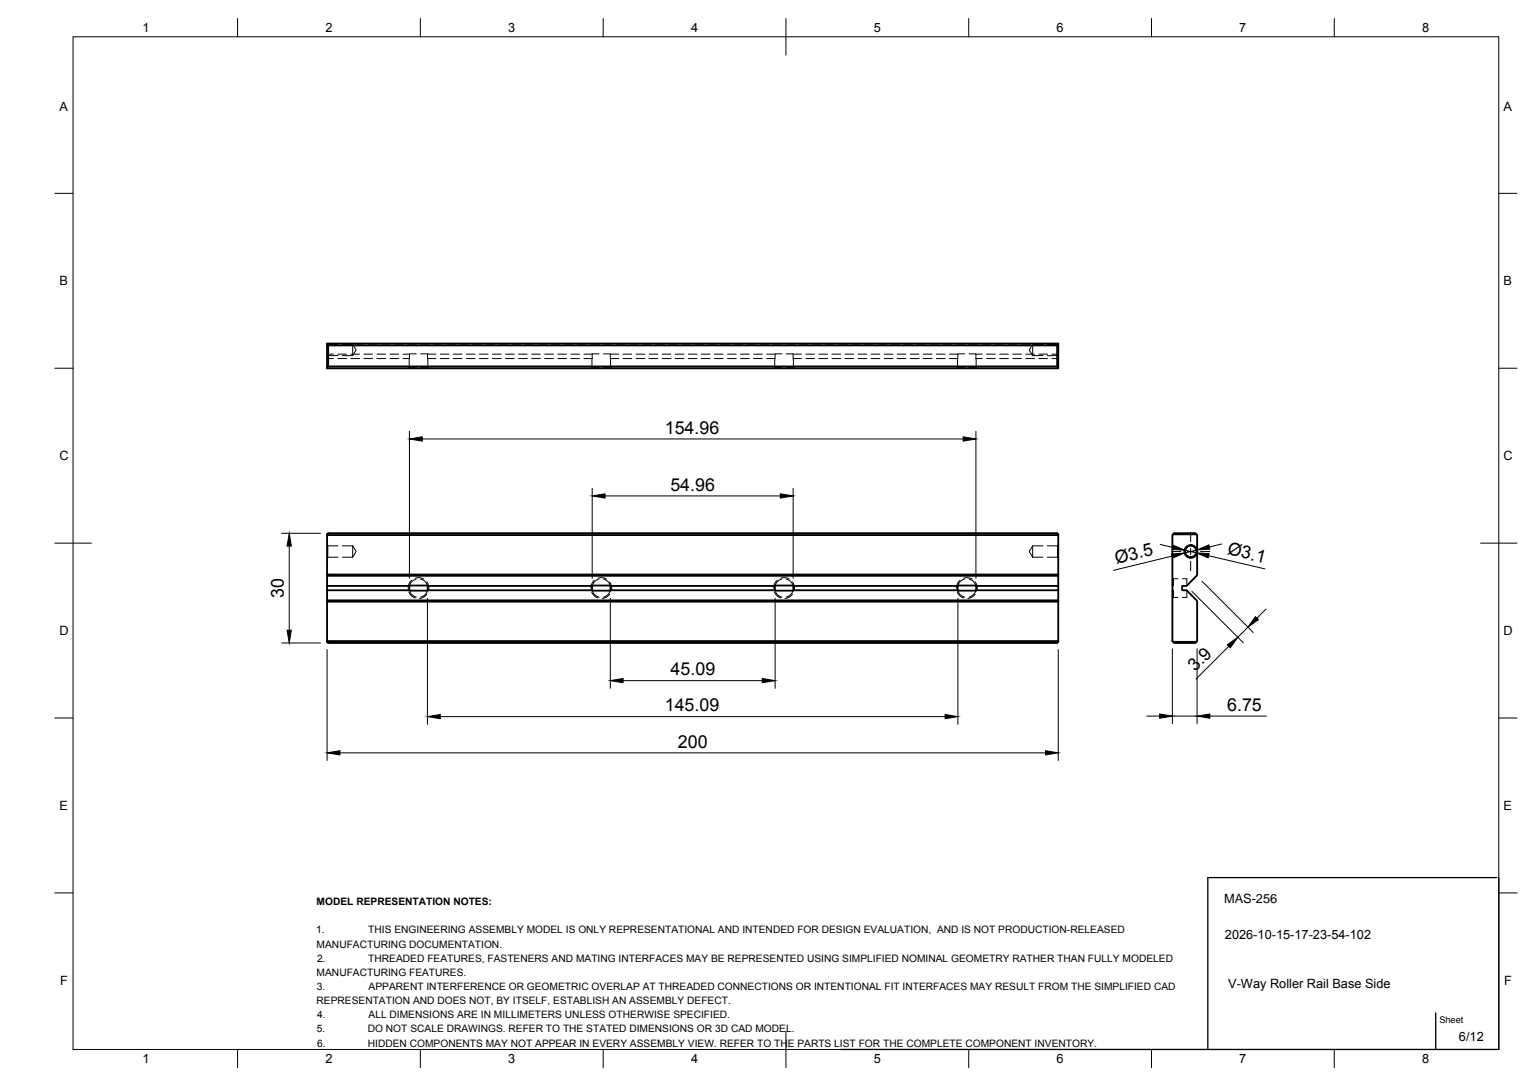
ISO-10303-21;
HEADER;
/* Generated by software containing ST-Developer
 * from STEP Tools, Inc. (www.steptools.com) 
 */

FILE_DESCRIPTION(
/* description */ (''),
/* implementation_level */ '2;1');

FILE_NAME(
/* name */ 'V-Way Roller Rail Base Side.step',
/* time_stamp */ '2026-10-14T18:40:07-07:00',
/* author */ (''),
/* organization */ (''),
/* preprocessor_version */ 'ST-DEVELOPER v20.2',
/* originating_system */ 'Autodesk Translation Framework v15.15.0.0',
/* authorisation */ '');

FILE_SCHEMA (('AUTOMOTIVE_DESIGN { 1 0 10303 214 3 1 1 }'));
ENDSEC;

DATA;
#10=MECHANICAL_DESIGN_GEOMETRIC_PRESENTATION_REPRESENTATION('',(#834),#81040);
#384=ELLIPSE('',#15733,3.60624458405138,2.54999999999999);
#385=ELLIPSE('',#15735,3.60624458405138,2.54999999999999);
#386=ELLIPSE('',#15737,3.60624458405138,2.54999999999999);
#387=ELLIPSE('',#15739,3.60624458405138,2.54999999999999);
#388=ELLIPSE('',#15745,3.60624458405139,2.55);
#389=ELLIPSE('',#15747,3.60624458405139,2.55);
#390=ELLIPSE('',#15749,3.60624458405139,2.55);
#391=ELLIPSE('',#15751,3.60624458405139,2.55);
#392=ELLIPSE('',#15757,3.60624458405141,2.55000000000001);
#393=ELLIPSE('',#15759,3.60624458405141,2.55000000000001);
#394=ELLIPSE('',#15761,3.6062445840514,2.55000000000001);
#395=ELLIPSE('',#15763,3.6062445840514,2.55000000000001);
#396=ELLIPSE('',#15769,3.60624458405141,2.55000000000001);
#397=ELLIPSE('',#15771,3.60624458405141,2.55000000000001);
#398=ELLIPSE('',#15773,3.6062445840514,2.55000000000001);
#399=ELLIPSE('',#15775,3.6062445840514,2.55000000000001);
#814=SHAPE_REPRESENTATION_RELATIONSHIP('SRR','None',#81133,#824);
#824=ADVANCED_BREP_SHAPE_REPRESENTATION('',(#844),#81033);
#834=STYLED_ITEM('',(#81192),#844);
#844=MANIFOLD_SOLID_BREP('Body1',#15087);
#920=CYLINDRICAL_SURFACE('',#15711,1.55);
#921=CYLINDRICAL_SURFACE('',#15720,1.55);
#922=CYLINDRICAL_SURFACE('',#15731,2.54999999999999);
#923=CYLINDRICAL_SURFACE('',#15743,2.55);
#924=CYLINDRICAL_SURFACE('',#15755,2.55000000000001);
#925=CYLINDRICAL_SURFACE('',#15767,2.55000000000001);
#1172=FACE_BOUND('',#2705,.T.);
#1173=FACE_BOUND('',#2706,.T.);
#1174=FACE_BOUND('',#2707,.T.);
#1175=FACE_BOUND('',#2708,.T.);
#1320=PLANE('',#15710);
#1321=PLANE('',#15719);
#1322=PLANE('',#15727);
#1323=PLANE('',#15777);
#1324=PLANE('',#15778);
#1325=PLANE('',#15779);
#1326=PLANE('',#15780);
#1327=PLANE('',#15781);
#1328=PLANE('',#15782);
#1329=PLANE('',#15783);
#1330=PLANE('',#15784);
#1331=PLANE('',#15785);
#1332=PLANE('',#15786);
#1333=PLANE('',#15787);
#1334=PLANE('',#15788);
#1335=PLANE('',#15789);
#1336=PLANE('',#15790);
#1337=PLANE('',#15791);
#1338=PLANE('',#15792);
#1339=PLANE('',#15793);
#1340=PLANE('',#15794);
#1341=PLANE('',#15795);
#1342=PLANE('',#15796);
#1343=PLANE('',#15797);
#1344=PLANE('',#15798);
#1345=PLANE('',#15799);
#1346=PLANE('',#15800);
#1347=PLANE('',#15801);
#1348=PLANE('',#15802);
#1349=PLANE('',#15803);
#1350=PLANE('',#15804);
#1351=PLANE('',#15805);
#1352=PLANE('',#15806);
#1353=PLANE('',#15807);
#1354=PLANE('',#15808);
#1355=PLANE('',#15809);
#1356=PLANE('',#15810);
#1357=PLANE('',#15811);
#1358=PLANE('',#15812);
#1359=PLANE('',#15813);
#1360=PLANE('',#15814);
#1361=PLANE('',#15815);
#1863=FACE_OUTER_BOUND('',#2695,.T.);
#1864=FACE_OUTER_BOUND('',#2696,.T.);
#1865=FACE_OUTER_BOUND('',#2697,.T.);
#1866=FACE_OUTER_BOUND('',#2698,.T.);
#1867=FACE_OUTER_BOUND('',#2699,.T.);
#1868=FACE_OUTER_BOUND('',#2700,.T.);
#1869=FACE_OUTER_BOUND('',#2701,.T.);
#1870=FACE_OUTER_BOUND('',#2702,.T.);
#1871=FACE_OUTER_BOUND('',#2703,.T.);
#1872=FACE_OUTER_BOUND('',#2704,.T.);
#1873=FACE_OUTER_BOUND('',#2709,.T.);
#1874=FACE_OUTER_BOUND('',#2710,.T.);
#1875=FACE_OUTER_BOUND('',#2711,.T.);
#1876=FACE_OUTER_BOUND('',#2712,.T.);
#1877=FACE_OUTER_BOUND('',#2713,.T.);
#1878=FACE_OUTER_BOUND('',#2714,.T.);
#1879=FACE_OUTER_BOUND('',#2715,.T.);
#1880=FACE_OUTER_BOUND('',#2716,.T.);
#1881=FACE_OUTER_BOUND('',#2717,.T.);
#1882=FACE_OUTER_BOUND('',#2718,.T.);
#1883=FACE_OUTER_BOUND('',#2719,.T.);
#1884=FACE_OUTER_BOUND('',#2720,.T.);
#1885=FACE_OUTER_BOUND('',#2721,.T.);
#1886=FACE_OUTER_BOUND('',#2722,.T.);
#1887=FACE_OUTER_BOUND('',#2723,.T.);
#1888=FACE_OUTER_BOUND('',#2724,.T.);
#1889=FACE_OUTER_BOUND('',#2725,.T.);
#1890=FACE_OUTER_BOUND('',#2726,.T.);
#1891=FACE_OUTER_BOUND('',#2727,.T.);
#1892=FACE_OUTER_BOUND('',#2728,.T.);
#1893=FACE_OUTER_BOUND('',#2729,.T.);
#1894=FACE_OUTER_BOUND('',#2730,.T.);
#1895=FACE_OUTER_BOUND('',#2731,.T.);
#1896=FACE_OUTER_BOUND('',#2732,.T.);
#1897=FACE_OUTER_BOUND('',#2733,.T.);
#1898=FACE_OUTER_BOUND('',#2734,.T.);
#1899=FACE_OUTER_BOUND('',#2735,.T.);
#1900=FACE_OUTER_BOUND('',#2736,.T.);
#1901=FACE_OUTER_BOUND('',#2737,.T.);
#1902=FACE_OUTER_BOUND('',#2738,.T.);
#1903=FACE_OUTER_BOUND('',#2739,.T.);
#1904=FACE_OUTER_BOUND('',#2740,.T.);
#1905=FACE_OUTER_BOUND('',#2741,.T.);
#1906=FACE_OUTER_BOUND('',#2742,.T.);
#1907=FACE_OUTER_BOUND('',#2743,.T.);
#1908=FACE_OUTER_BOUND('',#2744,.T.);
#1909=FACE_OUTER_BOUND('',#2745,.T.);
#1910=FACE_OUTER_BOUND('',#2746,.T.);
#1911=FACE_OUTER_BOUND('',#2747,.T.);
#1912=FACE_OUTER_BOUND('',#2748,.T.);
#1913=FACE_OUTER_BOUND('',#2749,.T.);
#1914=FACE_OUTER_BOUND('',#2750,.T.);
#1915=FACE_OUTER_BOUND('',#2751,.T.);
#1916=FACE_OUTER_BOUND('',#2752,.T.);
#1917=FACE_OUTER_BOUND('',#2753,.T.);
#1918=FACE_OUTER_BOUND('',#2754,.T.);
#2695=EDGE_LOOP('',(#11060,#11061,#11062,#11063,#11064));
#2696=EDGE_LOOP('',(#11065,#11066,#11067,#11068,#11069,#11070,#11071,#11072,
#11073,#11074,#11075,#11076,#11077,#11078,#11079,#11080,#11081,#11082,#11083));
#2697=EDGE_LOOP('',(#11084,#11085,#11086,#11087,#11088));
#2698=EDGE_LOOP('',(#11089,#11090,#11091,#11092));
#2699=EDGE_LOOP('',(#11093,#11094,#11095,#11096,#11097));
#2700=EDGE_LOOP('',(#11098,#11099,#11100,#11101,#11102,#11103,#11104,#11105,
#11106,#11107,#11108,#11109,#11110,#11111,#11112,#11113,#11114,#11115,#11116));
#2701=EDGE_LOOP('',(#11117,#11118,#11119,#11120,#11121));
#2702=EDGE_LOOP('',(#11122,#11123,#11124,#11125));
#2703=EDGE_LOOP('',(#11126,#11127,#11128,#11129));
#2704=EDGE_LOOP('',(#11130,#11131,#11132,#11133));
#2705=EDGE_LOOP('',(#11134));
#2706=EDGE_LOOP('',(#11135));
#2707=EDGE_LOOP('',(#11136));
#2708=EDGE_LOOP('',(#11137));
#2709=EDGE_LOOP('',(#11138,#11139,#11140,#11141,#11142,#11143,#11144,#11145,
#11146,#11147,#11148,#11149,#11150,#11151,#11152,#11153));
#2710=EDGE_LOOP('',(#11154,#11155,#11156,#11157));
#2711=EDGE_LOOP('',(#11158,#11159,#11160,#11161,#11162,#11163,#11164,#11165,
#11166,#11167,#11168,#11169,#11170,#11171,#11172,#11173));
#2712=EDGE_LOOP('',(#11174,#11175,#11176,#11177));
#2713=EDGE_LOOP('',(#11178,#11179,#11180,#11181,#11182,#11183,#11184,#11185,
#11186,#11187,#11188,#11189,#11190,#11191,#11192,#11193));
#2714=EDGE_LOOP('',(#11194,#11195,#11196,#11197));
#2715=EDGE_LOOP('',(#11198,#11199,#11200,#11201,#11202,#11203,#11204,#11205,
#11206,#11207,#11208,#11209,#11210,#11211,#11212,#11213));
#2716=EDGE_LOOP('',(#11214,#11215));
#2717=EDGE_LOOP('',(#11216,#11217));
#2718=EDGE_LOOP('',(#11218,#11219));
#2719=EDGE_LOOP('',(#11220,#11221));
#2720=EDGE_LOOP('',(#11222,#11223));
#2721=EDGE_LOOP('',(#11224,#11225));
#2722=EDGE_LOOP('',(#11226,#11227));
#2723=EDGE_LOOP('',(#11228,#11229));
#2724=EDGE_LOOP('',(#11230,#11231,#11232,#11233,#11234,#11235,#11236,#11237,
#11238,#11239,#11240,#11241,#11242,#11243,#11244,#11245,#11246,#11247,#11248,
#11249));
#2725=EDGE_LOOP('',(#11250,#11251,#11252,#11253));
#2726=EDGE_LOOP('',(#11254,#11255,#11256,#11257));
#2727=EDGE_LOOP('',(#11258,#11259,#11260,#11261));
#2728=EDGE_LOOP('',(#11262,#11263,#11264,#11265));
#2729=EDGE_LOOP('',(#11266,#11267,#11268,#11269));
#2730=EDGE_LOOP('',(#11270,#11271,#11272,#11273,#11274));
#2731=EDGE_LOOP('',(#11275,#11276,#11277,#11278,#11279));
#2732=EDGE_LOOP('',(#11280,#11281,#11282,#11283,#11284));
#2733=EDGE_LOOP('',(#11285,#11286,#11287,#11288));
#2734=EDGE_LOOP('',(#11289,#11290,#11291,#11292));
#2735=EDGE_LOOP('',(#11293,#11294,#11295,#11296));
#2736=EDGE_LOOP('',(#11297,#11298,#11299,#11300));
#2737=EDGE_LOOP('',(#11301,#11302,#11303,#11304));
#2738=EDGE_LOOP('',(#11305,#11306,#11307,#11308,#11309,#11310));
#2739=EDGE_LOOP('',(#11311,#11312,#11313,#11314));
#2740=EDGE_LOOP('',(#11315,#11316,#11317,#11318,#11319,#11320));
#2741=EDGE_LOOP('',(#11321,#11322,#11323,#11324));
#2742=EDGE_LOOP('',(#11325,#11326,#11327,#11328));
#2743=EDGE_LOOP('',(#11329,#11330,#11331,#11332));
#2744=EDGE_LOOP('',(#11333,#11334,#11335,#11336));
#2745=EDGE_LOOP('',(#11337,#11338,#11339,#11340));
#2746=EDGE_LOOP('',(#11341,#11342,#11343,#11344,#11345,#11346,#11347,#11348,
#11349,#11350,#11351,#11352,#11353,#11354,#11355,#11356,#11357,#11358,#11359,
#11360));
#2747=EDGE_LOOP('',(#11361,#11362,#11363,#11364));
#2748=EDGE_LOOP('',(#11365,#11366,#11367,#11368,#11369,#11370));
#2749=EDGE_LOOP('',(#11371,#11372,#11373,#11374,#11375,#11376));
#2750=EDGE_LOOP('',(#11377,#11378,#11379,#11380,#11381,#11382));
#2751=EDGE_LOOP('',(#11383,#11384,#11385,#11386));
#2752=EDGE_LOOP('',(#11387,#11388,#11389,#11390));
#2753=EDGE_LOOP('',(#11391,#11392,#11393,#11394,#11395));
#2754=EDGE_LOOP('',(#11396,#11397,#11398,#11399));
#3614=LINE('',#21912,#4726);
#3615=LINE('',#21919,#4727);
#3616=LINE('',#21921,#4728);
#3617=LINE('',#21923,#4729);
#3618=LINE('',#21925,#4730);
#3619=LINE('',#21927,#4731);
#3620=LINE('',#21929,#4732);
#3621=LINE('',#21931,#4733);
#3622=LINE('',#21933,#4734);
#3623=LINE('',#21935,#4735);
#3624=LINE('',#21937,#4736);
#3625=LINE('',#21938,#4737);
#3626=LINE('',#21940,#4738);
#3627=LINE('',#21942,#4739);
#3628=LINE('',#21944,#4740);
#3629=LINE('',#21946,#4741);
#3630=LINE('',#21948,#4742);
#3631=LINE('',#21949,#4743);
#3632=LINE('',#21952,#4744);
#3633=LINE('',#21958,#4745);
#3634=LINE('',#21963,#4746);
#3635=LINE('',#21970,#4747);
#3636=LINE('',#21972,#4748);
#3637=LINE('',#21973,#4749);
#3638=LINE('',#21975,#4750);
#3639=LINE('',#21977,#4751);
#3640=LINE('',#21979,#4752);
#3641=LINE('',#21981,#4753);
#3642=LINE('',#21983,#4754);
#3643=LINE('',#21985,#4755);
#3644=LINE('',#21987,#4756);
#3645=LINE('',#21989,#4757);
#3646=LINE('',#21991,#4758);
#3647=LINE('',#21993,#4759);
#3648=LINE('',#21995,#4760);
#3649=LINE('',#21997,#4761);
#3650=LINE('',#21999,#4762);
#3651=LINE('',#22000,#4763);
#3652=LINE('',#22003,#4764);
#3653=LINE('',#22009,#4765);
#3654=LINE('',#22014,#4766);
#3655=LINE('',#22017,#4767);
#3656=LINE('',#22018,#4768);
#3657=LINE('',#22027,#4769);
#3658=LINE('',#22031,#4770);
#3659=LINE('',#22039,#4771);
#3660=LINE('',#22043,#4772);
#3661=LINE('',#22051,#4773);
#3662=LINE('',#22056,#4774);
#3663=LINE('',#22059,#4775);
#3664=LINE('',#22063,#4776);
#3665=LINE('',#22071,#4777);
#3666=LINE('',#22075,#4778);
#3667=LINE('',#22083,#4779);
#3668=LINE('',#22088,#4780);
#3669=LINE('',#22091,#4781);
#3670=LINE('',#22095,#4782);
#3671=LINE('',#22103,#4783);
#3672=LINE('',#22107,#4784);
#3673=LINE('',#22115,#4785);
#3674=LINE('',#22120,#4786);
#3675=LINE('',#22123,#4787);
#3676=LINE('',#22127,#4788);
#3677=LINE('',#22135,#4789);
#3678=LINE('',#22139,#4790);
#3679=LINE('',#22147,#4791);
#3680=LINE('',#22150,#4792);
#3681=LINE('',#22152,#4793);
#3682=LINE('',#22154,#4794);
#3683=LINE('',#22156,#4795);
#3684=LINE('',#22158,#4796);
#3685=LINE('',#22160,#4797);
#3686=LINE('',#22162,#4798);
#3687=LINE('',#22164,#4799);
#3688=LINE('',#22166,#4800);
#3689=LINE('',#22167,#4801);
#3690=LINE('',#22168,#4802);
#3691=LINE('',#22169,#4803);
#3692=LINE('',#22170,#4804);
#3693=LINE('',#22171,#4805);
#3694=LINE('',#22173,#4806);
#3695=LINE('',#22175,#4807);
#3696=LINE('',#22177,#4808);
#3697=LINE('',#22179,#4809);
#3698=LINE('',#22181,#4810);
#3699=LINE('',#22183,#4811);
#3700=LINE('',#22185,#4812);
#3701=LINE('',#22187,#4813);
#3702=LINE('',#22189,#4814);
#3703=LINE('',#22191,#4815);
#3704=LINE('',#22193,#4816);
#3705=LINE('',#22195,#4817);
#3706=LINE('',#22198,#4818);
#3707=LINE('',#22200,#4819);
#3708=LINE('',#22201,#4820);
#3709=LINE('',#22204,#4821);
#3710=LINE('',#22205,#4822);
#3711=LINE('',#22208,#4823);
#3712=LINE('',#22210,#4824);
#3713=LINE('',#22211,#4825);
#3714=LINE('',#22214,#4826);
#3715=LINE('',#22215,#4827);
#3716=LINE('',#22218,#4828);
#3717=LINE('',#22219,#4829);
#3718=LINE('',#22222,#4830);
#3719=LINE('',#22223,#4831);
#3720=LINE('',#22225,#4832);
#3721=LINE('',#22227,#4833);
#3722=LINE('',#22229,#4834);
#3723=LINE('',#22230,#4835);
#3724=LINE('',#22232,#4836);
#3725=LINE('',#22234,#4837);
#3726=LINE('',#22237,#4838);
#3727=LINE('',#22238,#4839);
#3728=LINE('',#22242,#4840);
#3729=LINE('',#22244,#4841);
#4726=VECTOR('',#18020,1.65);
#4727=VECTOR('',#18027,10.);
#4728=VECTOR('',#18028,10.);
#4729=VECTOR('',#18029,10.);
#4730=VECTOR('',#18030,9.99999999999999);
#4731=VECTOR('',#18031,10.);
#4732=VECTOR('',#18032,10.);
#4733=VECTOR('',#18033,10.);
#4734=VECTOR('',#18034,10.);
#4735=VECTOR('',#18035,10.);
#4736=VECTOR('',#18036,9.99999999999999);
#4737=VECTOR('',#18037,10.);
#4738=VECTOR('',#18038,10.);
#4739=VECTOR('',#18039,10.);
#4740=VECTOR('',#18040,10.);
#4741=VECTOR('',#18041,10.);
#4742=VECTOR('',#18042,10.);
#4743=VECTOR('',#18043,10.);
#4744=VECTOR('',#18046,1.55);
#4745=VECTOR('',#18053,0.775000000000001);
#4746=VECTOR('',#18058,1.65);
#4747=VECTOR('',#18065,10.);
#4748=VECTOR('',#18066,10.);
#4749=VECTOR('',#18067,10.);
#4750=VECTOR('',#18068,10.);
#4751=VECTOR('',#18069,9.99999999999999);
#4752=VECTOR('',#18070,10.);
#4753=VECTOR('',#18071,10.);
#4754=VECTOR('',#18072,10.);
#4755=VECTOR('',#18073,10.);
#4756=VECTOR('',#18074,10.);
#4757=VECTOR('',#18075,9.99999999999999);
#4758=VECTOR('',#18076,10.);
#4759=VECTOR('',#18077,10.);
#4760=VECTOR('',#18078,10.);
#4761=VECTOR('',#18079,10.);
#4762=VECTOR('',#18080,10.);
#4763=VECTOR('',#18081,10.);
#4764=VECTOR('',#18084,1.55);
#4765=VECTOR('',#18091,1.55);
#4766=VECTOR('',#18096,2.7);
#4767=VECTOR('',#18101,10.);
#4768=VECTOR('',#18102,10.);
#4769=VECTOR('',#18111,2.54999999999999);
#4770=VECTOR('',#18114,10.);
#4771=VECTOR('',#18121,10.);
#4772=VECTOR('',#18124,10.);
#4773=VECTOR('',#18131,10.);
#4774=VECTOR('',#18138,2.7);
#4775=VECTOR('',#18141,2.55);
#4776=VECTOR('',#18144,10.);
#4777=VECTOR('',#18151,10.);
#4778=VECTOR('',#18154,10.);
#4779=VECTOR('',#18161,10.);
#4780=VECTOR('',#18168,2.7);
#4781=VECTOR('',#18171,2.55000000000001);
#4782=VECTOR('',#18174,10.);
#4783=VECTOR('',#18181,10.);
#4784=VECTOR('',#18184,10.);
#4785=VECTOR('',#18191,10.);
#4786=VECTOR('',#18198,2.7);
#4787=VECTOR('',#18201,2.55000000000001);
#4788=VECTOR('',#18204,10.);
#4789=VECTOR('',#18211,10.);
#4790=VECTOR('',#18214,10.);
#4791=VECTOR('',#18221,10.);
#4792=VECTOR('',#18226,10.);
#4793=VECTOR('',#18229,10.);
#4794=VECTOR('',#18232,10.);
#4795=VECTOR('',#18235,10.);
#4796=VECTOR('',#18238,10.);
#4797=VECTOR('',#18241,10.);
#4798=VECTOR('',#18244,10.);
#4799=VECTOR('',#18247,10.);
#4800=VECTOR('',#18250,10.);
#4801=VECTOR('',#18251,10.);
#4802=VECTOR('',#18252,10.);
#4803=VECTOR('',#18253,10.);
#4804=VECTOR('',#18254,10.);
#4805=VECTOR('',#18255,10.);
#4806=VECTOR('',#18258,10.);
#4807=VECTOR('',#18261,10.);
#4808=VECTOR('',#18264,10.);
#4809=VECTOR('',#18267,10.);
#4810=VECTOR('',#18270,10.);
#4811=VECTOR('',#18273,10.);
#4812=VECTOR('',#18276,10.);
#4813=VECTOR('',#18279,10.);
#4814=VECTOR('',#18282,10.);
#4815=VECTOR('',#18285,10.);
#4816=VECTOR('',#18288,10.);
#4817=VECTOR('',#18291,10.);
#4818=VECTOR('',#18294,10.);
#4819=VECTOR('',#18295,10.);
#4820=VECTOR('',#18296,10.);
#4821=VECTOR('',#18299,10.);
#4822=VECTOR('',#18300,10.);
#4823=VECTOR('',#18303,10.);
#4824=VECTOR('',#18304,10.);
#4825=VECTOR('',#18305,10.);
#4826=VECTOR('',#18308,10.);
#4827=VECTOR('',#18309,10.);
#4828=VECTOR('',#18312,10.);
#4829=VECTOR('',#18313,10.);
#4830=VECTOR('',#18316,10.);
#4831=VECTOR('',#18317,10.);
#4832=VECTOR('',#18320,10.);
#4833=VECTOR('',#18323,10.);
#4834=VECTOR('',#18326,10.);
#4835=VECTOR('',#18327,10.);
#4836=VECTOR('',#18330,10.);
#4837=VECTOR('',#18333,10.);
#4838=VECTOR('',#18338,10.);
#4839=VECTOR('',#18339,10.);
#4840=VECTOR('',#18346,10.);
#4841=VECTOR('',#18349,10.);
#5671=CIRCLE('',#15707,1.55);
#5672=CIRCLE('',#15708,1.75);
#5673=CIRCLE('',#15709,1.75);
#5674=CIRCLE('',#15712,1.55);
#5675=CIRCLE('',#15713,1.55);
#5676=CIRCLE('',#15716,1.55);
#5677=CIRCLE('',#15717,1.75);
#5678=CIRCLE('',#15718,1.75);
#5679=CIRCLE('',#15721,1.55);
#5680=CIRCLE('',#15722,1.55);
#5681=CIRCLE('',#15725,2.54999999999999);
#5682=CIRCLE('',#15726,2.85);
#5683=CIRCLE('',#15728,2.85);
#5684=CIRCLE('',#15729,2.85);
#5685=CIRCLE('',#15730,2.85);
#5686=CIRCLE('',#15732,2.54999999999999);
#5687=CIRCLE('',#15734,2.54999999999999);
#5688=CIRCLE('',#15736,2.54999999999999);
#5689=CIRCLE('',#15738,2.54999999999999);
#5690=CIRCLE('',#15740,2.54999999999999);
#5691=CIRCLE('',#15742,2.55);
#5692=CIRCLE('',#15744,2.55);
#5693=CIRCLE('',#15746,2.55);
#5694=CIRCLE('',#15748,2.55);
#5695=CIRCLE('',#15750,2.55);
#5696=CIRCLE('',#15752,2.55);
#5697=CIRCLE('',#15754,2.55000000000001);
#5698=CIRCLE('',#15756,2.55000000000001);
#5699=CIRCLE('',#15758,2.55000000000001);
#5700=CIRCLE('',#15760,2.55000000000001);
#5701=CIRCLE('',#15762,2.55000000000001);
#5702=CIRCLE('',#15764,2.55000000000001);
#5703=CIRCLE('',#15766,2.55000000000001);
#5704=CIRCLE('',#15768,2.55000000000001);
#5705=CIRCLE('',#15770,2.55000000000001);
#5706=CIRCLE('',#15772,2.55000000000001);
#5707=CIRCLE('',#15774,2.55000000000001);
#5708=CIRCLE('',#15776,2.55000000000001);
#6436=VERTEX_POINT('',#21909);
#6437=VERTEX_POINT('',#21911);
#6438=VERTEX_POINT('',#21913);
#6439=VERTEX_POINT('',#21917);
#6440=VERTEX_POINT('',#21918);
#6441=VERTEX_POINT('',#21920);
#6442=VERTEX_POINT('',#21922);
#6443=VERTEX_POINT('',#21924);
#6444=VERTEX_POINT('',#21926);
#6445=VERTEX_POINT('',#21928);
#6446=VERTEX_POINT('',#21930);
#6447=VERTEX_POINT('',#21932);
#6448=VERTEX_POINT('',#21934);
#6449=VERTEX_POINT('',#21936);
#6450=VERTEX_POINT('',#21939);
#6451=VERTEX_POINT('',#21941);
#6452=VERTEX_POINT('',#21943);
#6453=VERTEX_POINT('',#21945);
#6454=VERTEX_POINT('',#21947);
#6455=VERTEX_POINT('',#21951);
#6456=VERTEX_POINT('',#21953);
#6457=VERTEX_POINT('',#21957);
#6458=VERTEX_POINT('',#21960);
#6459=VERTEX_POINT('',#21962);
#6460=VERTEX_POINT('',#21964);
#6461=VERTEX_POINT('',#21968);
#6462=VERTEX_POINT('',#21969);
#6463=VERTEX_POINT('',#21971);
#6464=VERTEX_POINT('',#21974);
#6465=VERTEX_POINT('',#21976);
#6466=VERTEX_POINT('',#21978);
#6467=VERTEX_POINT('',#21980);
#6468=VERTEX_POINT('',#21982);
#6469=VERTEX_POINT('',#21984);
#6470=VERTEX_POINT('',#21986);
#6471=VERTEX_POINT('',#21988);
#6472=VERTEX_POINT('',#21990);
#6473=VERTEX_POINT('',#21992);
#6474=VERTEX_POINT('',#21994);
#6475=VERTEX_POINT('',#21996);
#6476=VERTEX_POINT('',#21998);
#6477=VERTEX_POINT('',#22002);
#6478=VERTEX_POINT('',#22004);
#6479=VERTEX_POINT('',#22008);
#6480=VERTEX_POINT('',#22011);
#6481=VERTEX_POINT('',#22013);
#6482=VERTEX_POINT('',#22019);
#6483=VERTEX_POINT('',#22021);
#6484=VERTEX_POINT('',#22023);
#6485=VERTEX_POINT('',#22026);
#6486=VERTEX_POINT('',#22028);
#6487=VERTEX_POINT('',#22030);
#6488=VERTEX_POINT('',#22032);
#6489=VERTEX_POINT('',#22034);
#6490=VERTEX_POINT('',#22036);
#6491=VERTEX_POINT('',#22038);
#6492=VERTEX_POINT('',#22040);
#6493=VERTEX_POINT('',#22042);
#6494=VERTEX_POINT('',#22044);
#6495=VERTEX_POINT('',#22046);
#6496=VERTEX_POINT('',#22048);
#6497=VERTEX_POINT('',#22050);
#6498=VERTEX_POINT('',#22054);
#6499=VERTEX_POINT('',#22058);
#6500=VERTEX_POINT('',#22060);
#6501=VERTEX_POINT('',#22062);
#6502=VERTEX_POINT('',#22064);
#6503=VERTEX_POINT('',#22066);
#6504=VERTEX_POINT('',#22068);
#6505=VERTEX_POINT('',#22070);
#6506=VERTEX_POINT('',#22072);
#6507=VERTEX_POINT('',#22074);
#6508=VERTEX_POINT('',#22076);
#6509=VERTEX_POINT('',#22078);
#6510=VERTEX_POINT('',#22080);
#6511=VERTEX_POINT('',#22082);
#6512=VERTEX_POINT('',#22086);
#6513=VERTEX_POINT('',#22090);
#6514=VERTEX_POINT('',#22092);
#6515=VERTEX_POINT('',#22094);
#6516=VERTEX_POINT('',#22096);
#6517=VERTEX_POINT('',#22098);
#6518=VERTEX_POINT('',#22100);
#6519=VERTEX_POINT('',#22102);
#6520=VERTEX_POINT('',#22104);
#6521=VERTEX_POINT('',#22106);
#6522=VERTEX_POINT('',#22108);
#6523=VERTEX_POINT('',#22110);
#6524=VERTEX_POINT('',#22112);
#6525=VERTEX_POINT('',#22114);
#6526=VERTEX_POINT('',#22118);
#6527=VERTEX_POINT('',#22122);
#6528=VERTEX_POINT('',#22124);
#6529=VERTEX_POINT('',#22126);
#6530=VERTEX_POINT('',#22128);
#6531=VERTEX_POINT('',#22130);
#6532=VERTEX_POINT('',#22132);
#6533=VERTEX_POINT('',#22134);
#6534=VERTEX_POINT('',#22136);
#6535=VERTEX_POINT('',#22138);
#6536=VERTEX_POINT('',#22140);
#6537=VERTEX_POINT('',#22142);
#6538=VERTEX_POINT('',#22144);
#6539=VERTEX_POINT('',#22146);
#6540=VERTEX_POINT('',#22197);
#6541=VERTEX_POINT('',#22199);
#6542=VERTEX_POINT('',#22203);
#6543=VERTEX_POINT('',#22207);
#6544=VERTEX_POINT('',#22209);
#6545=VERTEX_POINT('',#22213);
#6546=VERTEX_POINT('',#22217);
#6547=VERTEX_POINT('',#22221);
#8193=EDGE_CURVE('',#6436,#6436,#5671,.T.);
#8194=EDGE_CURVE('',#6436,#6437,#3614,.T.);
#8195=EDGE_CURVE('',#6437,#6438,#5672,.T.);
#8196=EDGE_CURVE('',#6438,#6437,#5673,.T.);
#8197=EDGE_CURVE('',#6439,#6440,#3615,.T.);
#8198=EDGE_CURVE('',#6441,#6439,#3616,.T.);
#8199=EDGE_CURVE('',#6441,#6442,#3617,.T.);
#8200=EDGE_CURVE('',#6443,#6442,#3618,.T.);
#8201=EDGE_CURVE('',#6443,#6444,#3619,.T.);
#8202=EDGE_CURVE('',#6444,#6445,#3620,.T.);
#8203=EDGE_CURVE('',#6445,#6446,#3621,.T.);
#8204=EDGE_CURVE('',#6446,#6447,#3622,.T.);
#8205=EDGE_CURVE('',#6447,#6448,#3623,.T.);
#8206=EDGE_CURVE('',#6449,#6448,#3624,.T.);
#8207=EDGE_CURVE('',#6449,#6438,#3625,.T.);
#8208=EDGE_CURVE('',#6438,#6450,#3626,.T.);
#8209=EDGE_CURVE('',#6451,#6450,#3627,.T.);
#8210=EDGE_CURVE('',#6452,#6451,#3628,.T.);
#8211=EDGE_CURVE('',#6453,#6452,#3629,.T.);
#8212=EDGE_CURVE('',#6453,#6454,#3630,.T.);
#8213=EDGE_CURVE('',#6440,#6454,#3631,.T.);
#8214=EDGE_CURVE('',#6436,#6455,#3632,.T.);
#8215=EDGE_CURVE('',#6455,#6456,#5674,.T.);
#8216=EDGE_CURVE('',#6456,#6455,#5675,.T.);
#8217=EDGE_CURVE('',#6457,#6456,#3633,.T.);
#8218=EDGE_CURVE('',#6458,#6458,#5676,.T.);
#8219=EDGE_CURVE('',#6458,#6459,#3634,.T.);
#8220=EDGE_CURVE('',#6459,#6460,#5677,.T.);
#8221=EDGE_CURVE('',#6460,#6459,#5678,.T.);
#8222=EDGE_CURVE('',#6461,#6462,#3635,.T.);
#8223=EDGE_CURVE('',#6463,#6461,#3636,.T.);
#8224=EDGE_CURVE('',#6460,#6463,#3637,.T.);
#8225=EDGE_CURVE('',#6464,#6460,#3638,.T.);
#8226=EDGE_CURVE('',#6465,#6464,#3639,.T.);
#8227=EDGE_CURVE('',#6466,#6465,#3640,.T.);
#8228=EDGE_CURVE('',#6467,#6466,#3641,.T.);
#8229=EDGE_CURVE('',#6468,#6467,#3642,.T.);
#8230=EDGE_CURVE('',#6469,#6468,#3643,.T.);
#8231=EDGE_CURVE('',#6470,#6469,#3644,.T.);
#8232=EDGE_CURVE('',#6471,#6470,#3645,.T.);
#8233=EDGE_CURVE('',#6472,#6471,#3646,.T.);
#8234=EDGE_CURVE('',#6473,#6472,#3647,.T.);
#8235=EDGE_CURVE('',#6474,#6473,#3648,.T.);
#8236=EDGE_CURVE('',#6475,#6474,#3649,.T.);
#8237=EDGE_CURVE('',#6476,#6475,#3650,.T.);
#8238=EDGE_CURVE('',#6462,#6476,#3651,.T.);
#8239=EDGE_CURVE('',#6458,#6477,#3652,.T.);
#8240=EDGE_CURVE('',#6477,#6478,#5679,.T.);
#8241=EDGE_CURVE('',#6478,#6477,#5680,.T.);
#8242=EDGE_CURVE('',#6479,#6478,#3653,.T.);
#8243=EDGE_CURVE('',#6480,#6480,#5681,.T.);
#8244=EDGE_CURVE('',#6480,#6481,#3654,.T.);
#8245=EDGE_CURVE('',#6481,#6481,#5682,.T.);
#8246=EDGE_CURVE('',#6454,#6475,#3655,.T.);
#8247=EDGE_CURVE('',#6476,#6453,#3656,.T.);
#8248=EDGE_CURVE('',#6482,#6482,#5683,.T.);
#8249=EDGE_CURVE('',#6483,#6483,#5684,.T.);
#8250=EDGE_CURVE('',#6484,#6484,#5685,.T.);
#8251=EDGE_CURVE('',#6480,#6485,#3657,.T.);
#8252=EDGE_CURVE('',#6486,#6485,#5686,.T.);
#8253=EDGE_CURVE('',#6487,#6486,#3658,.T.);
#8254=EDGE_CURVE('',#6488,#6487,#384,.T.);
#8255=EDGE_CURVE('',#6488,#6489,#5687,.T.);
#8256=EDGE_CURVE('',#6490,#6489,#385,.T.);
#8257=EDGE_CURVE('',#6491,#6490,#3659,.T.);
#8258=EDGE_CURVE('',#6492,#6491,#5688,.T.);
#8259=EDGE_CURVE('',#6493,#6492,#3660,.T.);
#8260=EDGE_CURVE('',#6494,#6493,#386,.T.);
#8261=EDGE_CURVE('',#6494,#6495,#5689,.T.);
#8262=EDGE_CURVE('',#6496,#6495,#387,.T.);
#8263=EDGE_CURVE('',#6497,#6496,#3661,.T.);
#8264=EDGE_CURVE('',#6485,#6497,#5690,.T.);
#8265=EDGE_CURVE('',#6498,#6498,#5691,.T.);
#8266=EDGE_CURVE('',#6498,#6482,#3662,.T.);
#8267=EDGE_CURVE('',#6498,#6499,#3663,.T.);
#8268=EDGE_CURVE('',#6500,#6499,#5692,.T.);
#8269=EDGE_CURVE('',#6501,#6500,#3664,.T.);
#8270=EDGE_CURVE('',#6502,#6501,#388,.T.);
#8271=EDGE_CURVE('',#6502,#6503,#5693,.T.);
#8272=EDGE_CURVE('',#6504,#6503,#389,.T.);
#8273=EDGE_CURVE('',#6505,#6504,#3665,.T.);
#8274=EDGE_CURVE('',#6506,#6505,#5694,.T.);
#8275=EDGE_CURVE('',#6507,#6506,#3666,.T.);
#8276=EDGE_CURVE('',#6508,#6507,#390,.T.);
#8277=EDGE_CURVE('',#6508,#6509,#5695,.T.);
#8278=EDGE_CURVE('',#6510,#6509,#391,.T.);
#8279=EDGE_CURVE('',#6511,#6510,#3667,.T.);
#8280=EDGE_CURVE('',#6499,#6511,#5696,.T.);
#8281=EDGE_CURVE('',#6512,#6512,#5697,.T.);
#8282=EDGE_CURVE('',#6512,#6484,#3668,.T.);
#8283=EDGE_CURVE('',#6512,#6513,#3669,.T.);
#8284=EDGE_CURVE('',#6514,#6513,#5698,.T.);
#8285=EDGE_CURVE('',#6515,#6514,#3670,.T.);
#8286=EDGE_CURVE('',#6516,#6515,#392,.T.);
#8287=EDGE_CURVE('',#6516,#6517,#5699,.T.);
#8288=EDGE_CURVE('',#6518,#6517,#393,.T.);
#8289=EDGE_CURVE('',#6519,#6518,#3671,.T.);
#8290=EDGE_CURVE('',#6520,#6519,#5700,.T.);
#8291=EDGE_CURVE('',#6521,#6520,#3672,.T.);
#8292=EDGE_CURVE('',#6522,#6521,#394,.T.);
#8293=EDGE_CURVE('',#6522,#6523,#5701,.T.);
#8294=EDGE_CURVE('',#6524,#6523,#395,.T.);
#8295=EDGE_CURVE('',#6525,#6524,#3673,.T.);
#8296=EDGE_CURVE('',#6513,#6525,#5702,.T.);
#8297=EDGE_CURVE('',#6526,#6526,#5703,.T.);
#8298=EDGE_CURVE('',#6526,#6483,#3674,.T.);
#8299=EDGE_CURVE('',#6526,#6527,#3675,.T.);
#8300=EDGE_CURVE('',#6528,#6527,#5704,.T.);
#8301=EDGE_CURVE('',#6529,#6528,#3676,.T.);
#8302=EDGE_CURVE('',#6530,#6529,#396,.T.);
#8303=EDGE_CURVE('',#6530,#6531,#5705,.T.);
#8304=EDGE_CURVE('',#6532,#6531,#397,.T.);
#8305=EDGE_CURVE('',#6533,#6532,#3677,.T.);
#8306=EDGE_CURVE('',#6534,#6533,#5706,.T.);
#8307=EDGE_CURVE('',#6535,#6534,#3678,.T.);
#8308=EDGE_CURVE('',#6536,#6535,#398,.T.);
#8309=EDGE_CURVE('',#6536,#6537,#5707,.T.);
#8310=EDGE_CURVE('',#6538,#6537,#399,.T.);
#8311=EDGE_CURVE('',#6539,#6538,#3679,.T.);
#8312=EDGE_CURVE('',#6527,#6539,#5708,.T.);
#8313=EDGE_CURVE('',#6531,#6530,#3680,.T.);
#8314=EDGE_CURVE('',#6537,#6536,#3681,.T.);
#8315=EDGE_CURVE('',#6517,#6516,#3682,.T.);
#8316=EDGE_CURVE('',#6523,#6522,#3683,.T.);
#8317=EDGE_CURVE('',#6503,#6502,#3684,.T.);
#8318=EDGE_CURVE('',#6509,#6508,#3685,.T.);
#8319=EDGE_CURVE('',#6489,#6488,#3686,.T.);
#8320=EDGE_CURVE('',#6495,#6494,#3687,.T.);
#8321=EDGE_CURVE('',#6535,#6496,#3688,.T.);
#8322=EDGE_CURVE('',#6493,#6444,#3689,.T.);
#8323=EDGE_CURVE('',#6470,#6443,#3690,.T.);
#8324=EDGE_CURVE('',#6469,#6510,#3691,.T.);
#8325=EDGE_CURVE('',#6507,#6524,#3692,.T.);
#8326=EDGE_CURVE('',#6521,#6538,#3693,.T.);
#8327=EDGE_CURVE('',#6492,#6445,#3694,.T.);
#8328=EDGE_CURVE('',#6534,#6497,#3695,.T.);
#8329=EDGE_CURVE('',#6468,#6511,#3696,.T.);
#8330=EDGE_CURVE('',#6506,#6525,#3697,.T.);
#8331=EDGE_CURVE('',#6491,#6446,#3698,.T.);
#8332=EDGE_CURVE('',#6533,#6486,#3699,.T.);
#8333=EDGE_CURVE('',#6467,#6500,#3700,.T.);
#8334=EDGE_CURVE('',#6505,#6514,#3701,.T.);
#8335=EDGE_CURVE('',#6490,#6447,#3702,.T.);
#8336=EDGE_CURVE('',#6532,#6487,#3703,.T.);
#8337=EDGE_CURVE('',#6466,#6501,#3704,.T.);
#8338=EDGE_CURVE('',#6504,#6515,#3705,.T.);
#8339=EDGE_CURVE('',#6540,#6439,#3706,.T.);
#8340=EDGE_CURVE('',#6440,#6541,#3707,.T.);
#8341=EDGE_CURVE('',#6541,#6540,#3708,.T.);
#8342=EDGE_CURVE('',#6542,#6474,#3709,.T.);
#8343=EDGE_CURVE('',#6542,#6541,#3710,.T.);
#8344=EDGE_CURVE('',#6543,#6452,#3711,.T.);
#8345=EDGE_CURVE('',#6451,#6544,#3712,.T.);
#8346=EDGE_CURVE('',#6544,#6543,#3713,.T.);
#8347=EDGE_CURVE('',#6543,#6545,#3714,.T.);
#8348=EDGE_CURVE('',#6462,#6545,#3715,.T.);
#8349=EDGE_CURVE('',#6545,#6546,#3716,.T.);
#8350=EDGE_CURVE('',#6546,#6461,#3717,.T.);
#8351=EDGE_CURVE('',#6473,#6547,#3718,.T.);
#8352=EDGE_CURVE('',#6547,#6542,#3719,.T.);
#8353=EDGE_CURVE('',#6442,#6471,#3720,.T.);
#8354=EDGE_CURVE('',#6472,#6441,#3721,.T.);
#8355=EDGE_CURVE('',#6448,#6465,#3722,.T.);
#8356=EDGE_CURVE('',#6464,#6449,#3723,.T.);
#8357=EDGE_CURVE('',#6518,#6529,#3724,.T.);
#8358=EDGE_CURVE('',#6540,#6547,#3725,.T.);
#8359=EDGE_CURVE('',#6450,#6463,#3726,.T.);
#8360=EDGE_CURVE('',#6546,#6544,#3727,.T.);
#8361=EDGE_CURVE('',#6519,#6528,#3728,.T.);
#8362=EDGE_CURVE('',#6520,#6539,#3729,.T.);
#11060=ORIENTED_EDGE('',*,*,#8193,.T.);
#11061=ORIENTED_EDGE('',*,*,#8194,.T.);
#11062=ORIENTED_EDGE('',*,*,#8195,.T.);
#11063=ORIENTED_EDGE('',*,*,#8196,.T.);
#11064=ORIENTED_EDGE('',*,*,#8194,.F.);
#11065=ORIENTED_EDGE('',*,*,#8197,.F.);
#11066=ORIENTED_EDGE('',*,*,#8198,.F.);
#11067=ORIENTED_EDGE('',*,*,#8199,.T.);
#11068=ORIENTED_EDGE('',*,*,#8200,.F.);
#11069=ORIENTED_EDGE('',*,*,#8201,.T.);
#11070=ORIENTED_EDGE('',*,*,#8202,.T.);
#11071=ORIENTED_EDGE('',*,*,#8203,.T.);
#11072=ORIENTED_EDGE('',*,*,#8204,.T.);
#11073=ORIENTED_EDGE('',*,*,#8205,.T.);
#11074=ORIENTED_EDGE('',*,*,#8206,.F.);
#11075=ORIENTED_EDGE('',*,*,#8207,.T.);
#11076=ORIENTED_EDGE('',*,*,#8195,.F.);
#11077=ORIENTED_EDGE('',*,*,#8196,.F.);
#11078=ORIENTED_EDGE('',*,*,#8208,.T.);
#11079=ORIENTED_EDGE('',*,*,#8209,.F.);
#11080=ORIENTED_EDGE('',*,*,#8210,.F.);
#11081=ORIENTED_EDGE('',*,*,#8211,.F.);
#11082=ORIENTED_EDGE('',*,*,#8212,.T.);
#11083=ORIENTED_EDGE('',*,*,#8213,.F.);
#11084=ORIENTED_EDGE('',*,*,#8193,.F.);
#11085=ORIENTED_EDGE('',*,*,#8214,.T.);
#11086=ORIENTED_EDGE('',*,*,#8215,.T.);
#11087=ORIENTED_EDGE('',*,*,#8216,.T.);
#11088=ORIENTED_EDGE('',*,*,#8214,.F.);
#11089=ORIENTED_EDGE('',*,*,#8217,.T.);
#11090=ORIENTED_EDGE('',*,*,#8215,.F.);
#11091=ORIENTED_EDGE('',*,*,#8216,.F.);
#11092=ORIENTED_EDGE('',*,*,#8217,.F.);
#11093=ORIENTED_EDGE('',*,*,#8218,.T.);
#11094=ORIENTED_EDGE('',*,*,#8219,.T.);
#11095=ORIENTED_EDGE('',*,*,#8220,.T.);
#11096=ORIENTED_EDGE('',*,*,#8221,.T.);
#11097=ORIENTED_EDGE('',*,*,#8219,.F.);
#11098=ORIENTED_EDGE('',*,*,#8222,.F.);
#11099=ORIENTED_EDGE('',*,*,#8223,.F.);
#11100=ORIENTED_EDGE('',*,*,#8224,.F.);
#11101=ORIENTED_EDGE('',*,*,#8220,.F.);
#11102=ORIENTED_EDGE('',*,*,#8221,.F.);
#11103=ORIENTED_EDGE('',*,*,#8225,.F.);
#11104=ORIENTED_EDGE('',*,*,#8226,.F.);
#11105=ORIENTED_EDGE('',*,*,#8227,.F.);
#11106=ORIENTED_EDGE('',*,*,#8228,.F.);
#11107=ORIENTED_EDGE('',*,*,#8229,.F.);
#11108=ORIENTED_EDGE('',*,*,#8230,.F.);
#11109=ORIENTED_EDGE('',*,*,#8231,.F.);
#11110=ORIENTED_EDGE('',*,*,#8232,.F.);
#11111=ORIENTED_EDGE('',*,*,#8233,.F.);
#11112=ORIENTED_EDGE('',*,*,#8234,.F.);
#11113=ORIENTED_EDGE('',*,*,#8235,.F.);
#11114=ORIENTED_EDGE('',*,*,#8236,.F.);
#11115=ORIENTED_EDGE('',*,*,#8237,.F.);
#11116=ORIENTED_EDGE('',*,*,#8238,.F.);
#11117=ORIENTED_EDGE('',*,*,#8218,.F.);
#11118=ORIENTED_EDGE('',*,*,#8239,.T.);
#11119=ORIENTED_EDGE('',*,*,#8240,.T.);
#11120=ORIENTED_EDGE('',*,*,#8241,.T.);
#11121=ORIENTED_EDGE('',*,*,#8239,.F.);
#11122=ORIENTED_EDGE('',*,*,#8242,.T.);
#11123=ORIENTED_EDGE('',*,*,#8240,.F.);
#11124=ORIENTED_EDGE('',*,*,#8241,.F.);
#11125=ORIENTED_EDGE('',*,*,#8242,.F.);
#11126=ORIENTED_EDGE('',*,*,#8243,.T.);
#11127=ORIENTED_EDGE('',*,*,#8244,.T.);
#11128=ORIENTED_EDGE('',*,*,#8245,.T.);
#11129=ORIENTED_EDGE('',*,*,#8244,.F.);
#11130=ORIENTED_EDGE('',*,*,#8246,.F.);
#11131=ORIENTED_EDGE('',*,*,#8212,.F.);
#11132=ORIENTED_EDGE('',*,*,#8247,.F.);
#11133=ORIENTED_EDGE('',*,*,#8237,.T.);
#11134=ORIENTED_EDGE('',*,*,#8248,.F.);
#11135=ORIENTED_EDGE('',*,*,#8249,.F.);
#11136=ORIENTED_EDGE('',*,*,#8250,.F.);
#11137=ORIENTED_EDGE('',*,*,#8245,.F.);
#11138=ORIENTED_EDGE('',*,*,#8243,.F.);
#11139=ORIENTED_EDGE('',*,*,#8251,.T.);
#11140=ORIENTED_EDGE('',*,*,#8252,.F.);
#11141=ORIENTED_EDGE('',*,*,#8253,.F.);
#11142=ORIENTED_EDGE('',*,*,#8254,.F.);
#11143=ORIENTED_EDGE('',*,*,#8255,.T.);
#11144=ORIENTED_EDGE('',*,*,#8256,.F.);
#11145=ORIENTED_EDGE('',*,*,#8257,.F.);
#11146=ORIENTED_EDGE('',*,*,#8258,.F.);
#11147=ORIENTED_EDGE('',*,*,#8259,.F.);
#11148=ORIENTED_EDGE('',*,*,#8260,.F.);
#11149=ORIENTED_EDGE('',*,*,#8261,.T.);
#11150=ORIENTED_EDGE('',*,*,#8262,.F.);
#11151=ORIENTED_EDGE('',*,*,#8263,.F.);
#11152=ORIENTED_EDGE('',*,*,#8264,.F.);
#11153=ORIENTED_EDGE('',*,*,#8251,.F.);
#11154=ORIENTED_EDGE('',*,*,#8265,.T.);
#11155=ORIENTED_EDGE('',*,*,#8266,.T.);
#11156=ORIENTED_EDGE('',*,*,#8248,.T.);
#11157=ORIENTED_EDGE('',*,*,#8266,.F.);
#11158=ORIENTED_EDGE('',*,*,#8265,.F.);
#11159=ORIENTED_EDGE('',*,*,#8267,.T.);
#11160=ORIENTED_EDGE('',*,*,#8268,.F.);
#11161=ORIENTED_EDGE('',*,*,#8269,.F.);
#11162=ORIENTED_EDGE('',*,*,#8270,.F.);
#11163=ORIENTED_EDGE('',*,*,#8271,.T.);
#11164=ORIENTED_EDGE('',*,*,#8272,.F.);
#11165=ORIENTED_EDGE('',*,*,#8273,.F.);
#11166=ORIENTED_EDGE('',*,*,#8274,.F.);
#11167=ORIENTED_EDGE('',*,*,#8275,.F.);
#11168=ORIENTED_EDGE('',*,*,#8276,.F.);
#11169=ORIENTED_EDGE('',*,*,#8277,.T.);
#11170=ORIENTED_EDGE('',*,*,#8278,.F.);
#11171=ORIENTED_EDGE('',*,*,#8279,.F.);
#11172=ORIENTED_EDGE('',*,*,#8280,.F.);
#11173=ORIENTED_EDGE('',*,*,#8267,.F.);
#11174=ORIENTED_EDGE('',*,*,#8281,.T.);
#11175=ORIENTED_EDGE('',*,*,#8282,.T.);
#11176=ORIENTED_EDGE('',*,*,#8250,.T.);
#11177=ORIENTED_EDGE('',*,*,#8282,.F.);
#11178=ORIENTED_EDGE('',*,*,#8281,.F.);
#11179=ORIENTED_EDGE('',*,*,#8283,.T.);
#11180=ORIENTED_EDGE('',*,*,#8284,.F.);
#11181=ORIENTED_EDGE('',*,*,#8285,.F.);
#11182=ORIENTED_EDGE('',*,*,#8286,.F.);
#11183=ORIENTED_EDGE('',*,*,#8287,.T.);
#11184=ORIENTED_EDGE('',*,*,#8288,.F.);
#11185=ORIENTED_EDGE('',*,*,#8289,.F.);
#11186=ORIENTED_EDGE('',*,*,#8290,.F.);
#11187=ORIENTED_EDGE('',*,*,#8291,.F.);
#11188=ORIENTED_EDGE('',*,*,#8292,.F.);
#11189=ORIENTED_EDGE('',*,*,#8293,.T.);
#11190=ORIENTED_EDGE('',*,*,#8294,.F.);
#11191=ORIENTED_EDGE('',*,*,#8295,.F.);
#11192=ORIENTED_EDGE('',*,*,#8296,.F.);
#11193=ORIENTED_EDGE('',*,*,#8283,.F.);
#11194=ORIENTED_EDGE('',*,*,#8297,.T.);
#11195=ORIENTED_EDGE('',*,*,#8298,.T.);
#11196=ORIENTED_EDGE('',*,*,#8249,.T.);
#11197=ORIENTED_EDGE('',*,*,#8298,.F.);
#11198=ORIENTED_EDGE('',*,*,#8297,.F.);
#11199=ORIENTED_EDGE('',*,*,#8299,.T.);
#11200=ORIENTED_EDGE('',*,*,#8300,.F.);
#11201=ORIENTED_EDGE('',*,*,#8301,.F.);
#11202=ORIENTED_EDGE('',*,*,#8302,.F.);
#11203=ORIENTED_EDGE('',*,*,#8303,.T.);
#11204=ORIENTED_EDGE('',*,*,#8304,.F.);
#11205=ORIENTED_EDGE('',*,*,#8305,.F.);
#11206=ORIENTED_EDGE('',*,*,#8306,.F.);
#11207=ORIENTED_EDGE('',*,*,#8307,.F.);
#11208=ORIENTED_EDGE('',*,*,#8308,.F.);
#11209=ORIENTED_EDGE('',*,*,#8309,.T.);
#11210=ORIENTED_EDGE('',*,*,#8310,.F.);
#11211=ORIENTED_EDGE('',*,*,#8311,.F.);
#11212=ORIENTED_EDGE('',*,*,#8312,.F.);
#11213=ORIENTED_EDGE('',*,*,#8299,.F.);
#11214=ORIENTED_EDGE('',*,*,#8313,.F.);
#11215=ORIENTED_EDGE('',*,*,#8303,.F.);
#11216=ORIENTED_EDGE('',*,*,#8314,.F.);
#11217=ORIENTED_EDGE('',*,*,#8309,.F.);
#11218=ORIENTED_EDGE('',*,*,#8315,.F.);
#11219=ORIENTED_EDGE('',*,*,#8287,.F.);
#11220=ORIENTED_EDGE('',*,*,#8316,.F.);
#11221=ORIENTED_EDGE('',*,*,#8293,.F.);
#11222=ORIENTED_EDGE('',*,*,#8317,.F.);
#11223=ORIENTED_EDGE('',*,*,#8271,.F.);
#11224=ORIENTED_EDGE('',*,*,#8318,.F.);
#11225=ORIENTED_EDGE('',*,*,#8277,.F.);
#11226=ORIENTED_EDGE('',*,*,#8319,.F.);
#11227=ORIENTED_EDGE('',*,*,#8255,.F.);
#11228=ORIENTED_EDGE('',*,*,#8320,.F.);
#11229=ORIENTED_EDGE('',*,*,#8261,.F.);
#11230=ORIENTED_EDGE('',*,*,#8310,.T.);
#11231=ORIENTED_EDGE('',*,*,#8314,.T.);
#11232=ORIENTED_EDGE('',*,*,#8308,.T.);
#11233=ORIENTED_EDGE('',*,*,#8321,.T.);
#11234=ORIENTED_EDGE('',*,*,#8262,.T.);
#11235=ORIENTED_EDGE('',*,*,#8320,.T.);
#11236=ORIENTED_EDGE('',*,*,#8260,.T.);
#11237=ORIENTED_EDGE('',*,*,#8322,.T.);
#11238=ORIENTED_EDGE('',*,*,#8201,.F.);
#11239=ORIENTED_EDGE('',*,*,#8323,.F.);
#11240=ORIENTED_EDGE('',*,*,#8231,.T.);
#11241=ORIENTED_EDGE('',*,*,#8324,.T.);
#11242=ORIENTED_EDGE('',*,*,#8278,.T.);
#11243=ORIENTED_EDGE('',*,*,#8318,.T.);
#11244=ORIENTED_EDGE('',*,*,#8276,.T.);
#11245=ORIENTED_EDGE('',*,*,#8325,.T.);
#11246=ORIENTED_EDGE('',*,*,#8294,.T.);
#11247=ORIENTED_EDGE('',*,*,#8316,.T.);
#11248=ORIENTED_EDGE('',*,*,#8292,.T.);
#11249=ORIENTED_EDGE('',*,*,#8326,.T.);
#11250=ORIENTED_EDGE('',*,*,#8259,.T.);
#11251=ORIENTED_EDGE('',*,*,#8327,.T.);
#11252=ORIENTED_EDGE('',*,*,#8202,.F.);
#11253=ORIENTED_EDGE('',*,*,#8322,.F.);
#11254=ORIENTED_EDGE('',*,*,#8307,.T.);
#11255=ORIENTED_EDGE('',*,*,#8328,.T.);
#11256=ORIENTED_EDGE('',*,*,#8263,.T.);
#11257=ORIENTED_EDGE('',*,*,#8321,.F.);
#11258=ORIENTED_EDGE('',*,*,#8279,.T.);
#11259=ORIENTED_EDGE('',*,*,#8324,.F.);
#11260=ORIENTED_EDGE('',*,*,#8230,.T.);
#11261=ORIENTED_EDGE('',*,*,#8329,.T.);
#11262=ORIENTED_EDGE('',*,*,#8295,.T.);
#11263=ORIENTED_EDGE('',*,*,#8325,.F.);
#11264=ORIENTED_EDGE('',*,*,#8275,.T.);
#11265=ORIENTED_EDGE('',*,*,#8330,.T.);
#11266=ORIENTED_EDGE('',*,*,#8258,.T.);
#11267=ORIENTED_EDGE('',*,*,#8331,.T.);
#11268=ORIENTED_EDGE('',*,*,#8203,.F.);
#11269=ORIENTED_EDGE('',*,*,#8327,.F.);
#11270=ORIENTED_EDGE('',*,*,#8306,.T.);
#11271=ORIENTED_EDGE('',*,*,#8332,.T.);
#11272=ORIENTED_EDGE('',*,*,#8252,.T.);
#11273=ORIENTED_EDGE('',*,*,#8264,.T.);
#11274=ORIENTED_EDGE('',*,*,#8328,.F.);
#11275=ORIENTED_EDGE('',*,*,#8268,.T.);
#11276=ORIENTED_EDGE('',*,*,#8280,.T.);
#11277=ORIENTED_EDGE('',*,*,#8329,.F.);
#11278=ORIENTED_EDGE('',*,*,#8229,.T.);
#11279=ORIENTED_EDGE('',*,*,#8333,.T.);
#11280=ORIENTED_EDGE('',*,*,#8284,.T.);
#11281=ORIENTED_EDGE('',*,*,#8296,.T.);
#11282=ORIENTED_EDGE('',*,*,#8330,.F.);
#11283=ORIENTED_EDGE('',*,*,#8274,.T.);
#11284=ORIENTED_EDGE('',*,*,#8334,.T.);
#11285=ORIENTED_EDGE('',*,*,#8257,.T.);
#11286=ORIENTED_EDGE('',*,*,#8335,.T.);
#11287=ORIENTED_EDGE('',*,*,#8204,.F.);
#11288=ORIENTED_EDGE('',*,*,#8331,.F.);
#11289=ORIENTED_EDGE('',*,*,#8305,.T.);
#11290=ORIENTED_EDGE('',*,*,#8336,.T.);
#11291=ORIENTED_EDGE('',*,*,#8253,.T.);
#11292=ORIENTED_EDGE('',*,*,#8332,.F.);
#11293=ORIENTED_EDGE('',*,*,#8269,.T.);
#11294=ORIENTED_EDGE('',*,*,#8333,.F.);
#11295=ORIENTED_EDGE('',*,*,#8228,.T.);
#11296=ORIENTED_EDGE('',*,*,#8337,.T.);
#11297=ORIENTED_EDGE('',*,*,#8285,.T.);
#11298=ORIENTED_EDGE('',*,*,#8334,.F.);
#11299=ORIENTED_EDGE('',*,*,#8273,.T.);
#11300=ORIENTED_EDGE('',*,*,#8338,.T.);
#11301=ORIENTED_EDGE('',*,*,#8339,.T.);
#11302=ORIENTED_EDGE('',*,*,#8197,.T.);
#11303=ORIENTED_EDGE('',*,*,#8340,.T.);
#11304=ORIENTED_EDGE('',*,*,#8341,.T.);
#11305=ORIENTED_EDGE('',*,*,#8340,.F.);
#11306=ORIENTED_EDGE('',*,*,#8213,.T.);
#11307=ORIENTED_EDGE('',*,*,#8246,.T.);
#11308=ORIENTED_EDGE('',*,*,#8236,.T.);
#11309=ORIENTED_EDGE('',*,*,#8342,.F.);
#11310=ORIENTED_EDGE('',*,*,#8343,.T.);
#11311=ORIENTED_EDGE('',*,*,#8344,.T.);
#11312=ORIENTED_EDGE('',*,*,#8210,.T.);
#11313=ORIENTED_EDGE('',*,*,#8345,.T.);
#11314=ORIENTED_EDGE('',*,*,#8346,.T.);
#11315=ORIENTED_EDGE('',*,*,#8344,.F.);
#11316=ORIENTED_EDGE('',*,*,#8347,.T.);
#11317=ORIENTED_EDGE('',*,*,#8348,.F.);
#11318=ORIENTED_EDGE('',*,*,#8238,.T.);
#11319=ORIENTED_EDGE('',*,*,#8247,.T.);
#11320=ORIENTED_EDGE('',*,*,#8211,.T.);
#11321=ORIENTED_EDGE('',*,*,#8348,.T.);
#11322=ORIENTED_EDGE('',*,*,#8349,.T.);
#11323=ORIENTED_EDGE('',*,*,#8350,.T.);
#11324=ORIENTED_EDGE('',*,*,#8222,.T.);
#11325=ORIENTED_EDGE('',*,*,#8351,.T.);
#11326=ORIENTED_EDGE('',*,*,#8352,.T.);
#11327=ORIENTED_EDGE('',*,*,#8342,.T.);
#11328=ORIENTED_EDGE('',*,*,#8235,.T.);
#11329=ORIENTED_EDGE('',*,*,#8200,.T.);
#11330=ORIENTED_EDGE('',*,*,#8353,.T.);
#11331=ORIENTED_EDGE('',*,*,#8232,.T.);
#11332=ORIENTED_EDGE('',*,*,#8323,.T.);
#11333=ORIENTED_EDGE('',*,*,#8353,.F.);
#11334=ORIENTED_EDGE('',*,*,#8199,.F.);
#11335=ORIENTED_EDGE('',*,*,#8354,.F.);
#11336=ORIENTED_EDGE('',*,*,#8233,.T.);
#11337=ORIENTED_EDGE('',*,*,#8206,.T.);
#11338=ORIENTED_EDGE('',*,*,#8355,.T.);
#11339=ORIENTED_EDGE('',*,*,#8226,.T.);
#11340=ORIENTED_EDGE('',*,*,#8356,.T.);
#11341=ORIENTED_EDGE('',*,*,#8302,.T.);
#11342=ORIENTED_EDGE('',*,*,#8357,.F.);
#11343=ORIENTED_EDGE('',*,*,#8288,.T.);
#11344=ORIENTED_EDGE('',*,*,#8315,.T.);
#11345=ORIENTED_EDGE('',*,*,#8286,.T.);
#11346=ORIENTED_EDGE('',*,*,#8338,.F.);
#11347=ORIENTED_EDGE('',*,*,#8272,.T.);
#11348=ORIENTED_EDGE('',*,*,#8317,.T.);
#11349=ORIENTED_EDGE('',*,*,#8270,.T.);
#11350=ORIENTED_EDGE('',*,*,#8337,.F.);
#11351=ORIENTED_EDGE('',*,*,#8227,.T.);
#11352=ORIENTED_EDGE('',*,*,#8355,.F.);
#11353=ORIENTED_EDGE('',*,*,#8205,.F.);
#11354=ORIENTED_EDGE('',*,*,#8335,.F.);
#11355=ORIENTED_EDGE('',*,*,#8256,.T.);
#11356=ORIENTED_EDGE('',*,*,#8319,.T.);
#11357=ORIENTED_EDGE('',*,*,#8254,.T.);
#11358=ORIENTED_EDGE('',*,*,#8336,.F.);
#11359=ORIENTED_EDGE('',*,*,#8304,.T.);
#11360=ORIENTED_EDGE('',*,*,#8313,.T.);
#11361=ORIENTED_EDGE('',*,*,#8341,.F.);
#11362=ORIENTED_EDGE('',*,*,#8343,.F.);
#11363=ORIENTED_EDGE('',*,*,#8352,.F.);
#11364=ORIENTED_EDGE('',*,*,#8358,.F.);
#11365=ORIENTED_EDGE('',*,*,#8339,.F.);
#11366=ORIENTED_EDGE('',*,*,#8358,.T.);
#11367=ORIENTED_EDGE('',*,*,#8351,.F.);
#11368=ORIENTED_EDGE('',*,*,#8234,.T.);
#11369=ORIENTED_EDGE('',*,*,#8354,.T.);
#11370=ORIENTED_EDGE('',*,*,#8198,.T.);
#11371=ORIENTED_EDGE('',*,*,#8345,.F.);
#11372=ORIENTED_EDGE('',*,*,#8209,.T.);
#11373=ORIENTED_EDGE('',*,*,#8359,.T.);
#11374=ORIENTED_EDGE('',*,*,#8223,.T.);
#11375=ORIENTED_EDGE('',*,*,#8350,.F.);
#11376=ORIENTED_EDGE('',*,*,#8360,.T.);
#11377=ORIENTED_EDGE('',*,*,#8356,.F.);
#11378=ORIENTED_EDGE('',*,*,#8225,.T.);
#11379=ORIENTED_EDGE('',*,*,#8224,.T.);
#11380=ORIENTED_EDGE('',*,*,#8359,.F.);
#11381=ORIENTED_EDGE('',*,*,#8208,.F.);
#11382=ORIENTED_EDGE('',*,*,#8207,.F.);
#11383=ORIENTED_EDGE('',*,*,#8346,.F.);
#11384=ORIENTED_EDGE('',*,*,#8360,.F.);
#11385=ORIENTED_EDGE('',*,*,#8349,.F.);
#11386=ORIENTED_EDGE('',*,*,#8347,.F.);
#11387=ORIENTED_EDGE('',*,*,#8301,.T.);
#11388=ORIENTED_EDGE('',*,*,#8361,.F.);
#11389=ORIENTED_EDGE('',*,*,#8289,.T.);
#11390=ORIENTED_EDGE('',*,*,#8357,.T.);
#11391=ORIENTED_EDGE('',*,*,#8300,.T.);
#11392=ORIENTED_EDGE('',*,*,#8312,.T.);
#11393=ORIENTED_EDGE('',*,*,#8362,.F.);
#11394=ORIENTED_EDGE('',*,*,#8290,.T.);
#11395=ORIENTED_EDGE('',*,*,#8361,.T.);
#11396=ORIENTED_EDGE('',*,*,#8311,.T.);
#11397=ORIENTED_EDGE('',*,*,#8326,.F.);
#11398=ORIENTED_EDGE('',*,*,#8291,.T.);
#11399=ORIENTED_EDGE('',*,*,#8362,.T.);
#14317=CONICAL_SURFACE('',#15706,1.65,0.785398163397459);
#14318=CONICAL_SURFACE('',#15714,0.775000000000001,1.02974425867665);
#14319=CONICAL_SURFACE('',#15715,1.65,0.785398163397448);
#14320=CONICAL_SURFACE('',#15723,1.55,1.02974425867665);
#14321=CONICAL_SURFACE('',#15724,2.7,0.785398163397471);
#14322=CONICAL_SURFACE('',#15741,2.7,0.785398163397448);
#14323=CONICAL_SURFACE('',#15753,2.7,0.785398163397441);
#14324=CONICAL_SURFACE('',#15765,2.7,0.785398163397441);
#14598=ADVANCED_FACE('',(#1863),#14317,.F.);
#14599=ADVANCED_FACE('',(#1864),#1320,.T.);
#14600=ADVANCED_FACE('',(#1865),#920,.F.);
#14601=ADVANCED_FACE('',(#1866),#14318,.F.);
#14602=ADVANCED_FACE('',(#1867),#14319,.F.);
#14603=ADVANCED_FACE('',(#1868),#1321,.F.);
#14604=ADVANCED_FACE('',(#1869),#921,.F.);
#14605=ADVANCED_FACE('',(#1870),#14320,.F.);
#14606=ADVANCED_FACE('',(#1871),#14321,.F.);
#14607=ADVANCED_FACE('',(#1872,#1172,#1173,#1174,#1175),#1322,.T.);
#14608=ADVANCED_FACE('',(#1873),#922,.F.);
#14609=ADVANCED_FACE('',(#1874),#14322,.F.);
#14610=ADVANCED_FACE('',(#1875),#923,.F.);
#14611=ADVANCED_FACE('',(#1876),#14323,.F.);
#14612=ADVANCED_FACE('',(#1877),#924,.F.);
#14613=ADVANCED_FACE('',(#1878),#14324,.F.);
#14614=ADVANCED_FACE('',(#1879),#925,.F.);
#14615=ADVANCED_FACE('',(#1880),#1323,.T.);
#14616=ADVANCED_FACE('',(#1881),#1324,.T.);
#14617=ADVANCED_FACE('',(#1882),#1325,.T.);
#14618=ADVANCED_FACE('',(#1883),#1326,.T.);
#14619=ADVANCED_FACE('',(#1884),#1327,.T.);
#14620=ADVANCED_FACE('',(#1885),#1328,.T.);
#14621=ADVANCED_FACE('',(#1886),#1329,.T.);
#14622=ADVANCED_FACE('',(#1887),#1330,.T.);
#14623=ADVANCED_FACE('',(#1888),#1331,.T.);
#14624=ADVANCED_FACE('',(#1889),#1332,.T.);
#14625=ADVANCED_FACE('',(#1890),#1333,.T.);
#14626=ADVANCED_FACE('',(#1891),#1334,.T.);
#14627=ADVANCED_FACE('',(#1892),#1335,.T.);
#14628=ADVANCED_FACE('',(#1893),#1336,.T.);
#14629=ADVANCED_FACE('',(#1894),#1337,.T.);
#14630=ADVANCED_FACE('',(#1895),#1338,.T.);
#14631=ADVANCED_FACE('',(#1896),#1339,.T.);
#14632=ADVANCED_FACE('',(#1897),#1340,.T.);
#14633=ADVANCED_FACE('',(#1898),#1341,.T.);
#14634=ADVANCED_FACE('',(#1899),#1342,.T.);
#14635=ADVANCED_FACE('',(#1900),#1343,.T.);
#14636=ADVANCED_FACE('',(#1901),#1344,.T.);
#14637=ADVANCED_FACE('',(#1902),#1345,.T.);
#14638=ADVANCED_FACE('',(#1903),#1346,.T.);
#14639=ADVANCED_FACE('',(#1904),#1347,.T.);
#14640=ADVANCED_FACE('',(#1905),#1348,.T.);
#14641=ADVANCED_FACE('',(#1906),#1349,.T.);
#14642=ADVANCED_FACE('',(#1907),#1350,.T.);
#14643=ADVANCED_FACE('',(#1908),#1351,.T.);
#14644=ADVANCED_FACE('',(#1909),#1352,.T.);
#14645=ADVANCED_FACE('',(#1910),#1353,.T.);
#14646=ADVANCED_FACE('',(#1911),#1354,.T.);
#14647=ADVANCED_FACE('',(#1912),#1355,.T.);
#14648=ADVANCED_FACE('',(#1913),#1356,.T.);
#14649=ADVANCED_FACE('',(#1914),#1357,.T.);
#14650=ADVANCED_FACE('',(#1915),#1358,.T.);
#14651=ADVANCED_FACE('',(#1916),#1359,.T.);
#14652=ADVANCED_FACE('',(#1917),#1360,.T.);
#14653=ADVANCED_FACE('',(#1918),#1361,.T.);
#15087=CLOSED_SHELL('',(#14598,#14599,#14600,#14601,#14602,#14603,#14604,
#14605,#14606,#14607,#14608,#14609,#14610,#14611,#14612,#14613,#14614,#14615,
#14616,#14617,#14618,#14619,#14620,#14621,#14622,#14623,#14624,#14625,#14626,
#14627,#14628,#14629,#14630,#14631,#14632,#14633,#14634,#14635,#14636,#14637,
#14638,#14639,#14640,#14641,#14642,#14643,#14644,#14645,#14646,#14647,#14648,
#14649,#14650,#14651,#14652,#14653));
#15705=AXIS2_PLACEMENT_3D('',#21907,#18014,#18015);
#15706=AXIS2_PLACEMENT_3D('',#21908,#18016,#18017);
#15707=AXIS2_PLACEMENT_3D('',#21910,#18018,#18019);
#15708=AXIS2_PLACEMENT_3D('',#21914,#18021,#18022);
#15709=AXIS2_PLACEMENT_3D('',#21915,#18023,#18024);
#15710=AXIS2_PLACEMENT_3D('',#21916,#18025,#18026);
#15711=AXIS2_PLACEMENT_3D('',#21950,#18044,#18045);
#15712=AXIS2_PLACEMENT_3D('',#21954,#18047,#18048);
#15713=AXIS2_PLACEMENT_3D('',#21955,#18049,#18050);
#15714=AXIS2_PLACEMENT_3D('',#21956,#18051,#18052);
#15715=AXIS2_PLACEMENT_3D('',#21959,#18054,#18055);
#15716=AXIS2_PLACEMENT_3D('',#21961,#18056,#18057);
#15717=AXIS2_PLACEMENT_3D('',#21965,#18059,#18060);
#15718=AXIS2_PLACEMENT_3D('',#21966,#18061,#18062);
#15719=AXIS2_PLACEMENT_3D('',#21967,#18063,#18064);
#15720=AXIS2_PLACEMENT_3D('',#22001,#18082,#18083);
#15721=AXIS2_PLACEMENT_3D('',#22005,#18085,#18086);
#15722=AXIS2_PLACEMENT_3D('',#22006,#18087,#18088);
#15723=AXIS2_PLACEMENT_3D('',#22007,#18089,#18090);
#15724=AXIS2_PLACEMENT_3D('',#22010,#18092,#18093);
#15725=AXIS2_PLACEMENT_3D('',#22012,#18094,#18095);
#15726=AXIS2_PLACEMENT_3D('',#22015,#18097,#18098);
#15727=AXIS2_PLACEMENT_3D('',#22016,#18099,#18100);
#15728=AXIS2_PLACEMENT_3D('',#22020,#18103,#18104);
#15729=AXIS2_PLACEMENT_3D('',#22022,#18105,#18106);
#15730=AXIS2_PLACEMENT_3D('',#22024,#18107,#18108);
#15731=AXIS2_PLACEMENT_3D('',#22025,#18109,#18110);
#15732=AXIS2_PLACEMENT_3D('',#22029,#18112,#18113);
#15733=AXIS2_PLACEMENT_3D('',#22033,#18115,#18116);
#15734=AXIS2_PLACEMENT_3D('',#22035,#18117,#18118);
#15735=AXIS2_PLACEMENT_3D('',#22037,#18119,#18120);
#15736=AXIS2_PLACEMENT_3D('',#22041,#18122,#18123);
#15737=AXIS2_PLACEMENT_3D('',#22045,#18125,#18126);
#15738=AXIS2_PLACEMENT_3D('',#22047,#18127,#18128);
#15739=AXIS2_PLACEMENT_3D('',#22049,#18129,#18130);
#15740=AXIS2_PLACEMENT_3D('',#22052,#18132,#18133);
#15741=AXIS2_PLACEMENT_3D('',#22053,#18134,#18135);
#15742=AXIS2_PLACEMENT_3D('',#22055,#18136,#18137);
#15743=AXIS2_PLACEMENT_3D('',#22057,#18139,#18140);
#15744=AXIS2_PLACEMENT_3D('',#22061,#18142,#18143);
#15745=AXIS2_PLACEMENT_3D('',#22065,#18145,#18146);
#15746=AXIS2_PLACEMENT_3D('',#22067,#18147,#18148);
#15747=AXIS2_PLACEMENT_3D('',#22069,#18149,#18150);
#15748=AXIS2_PLACEMENT_3D('',#22073,#18152,#18153);
#15749=AXIS2_PLACEMENT_3D('',#22077,#18155,#18156);
#15750=AXIS2_PLACEMENT_3D('',#22079,#18157,#18158);
#15751=AXIS2_PLACEMENT_3D('',#22081,#18159,#18160);
#15752=AXIS2_PLACEMENT_3D('',#22084,#18162,#18163);
#15753=AXIS2_PLACEMENT_3D('',#22085,#18164,#18165);
#15754=AXIS2_PLACEMENT_3D('',#22087,#18166,#18167);
#15755=AXIS2_PLACEMENT_3D('',#22089,#18169,#18170);
#15756=AXIS2_PLACEMENT_3D('',#22093,#18172,#18173);
#15757=AXIS2_PLACEMENT_3D('',#22097,#18175,#18176);
#15758=AXIS2_PLACEMENT_3D('',#22099,#18177,#18178);
#15759=AXIS2_PLACEMENT_3D('',#22101,#18179,#18180);
#15760=AXIS2_PLACEMENT_3D('',#22105,#18182,#18183);
#15761=AXIS2_PLACEMENT_3D('',#22109,#18185,#18186);
#15762=AXIS2_PLACEMENT_3D('',#22111,#18187,#18188);
#15763=AXIS2_PLACEMENT_3D('',#22113,#18189,#18190);
#15764=AXIS2_PLACEMENT_3D('',#22116,#18192,#18193);
#15765=AXIS2_PLACEMENT_3D('',#22117,#18194,#18195);
#15766=AXIS2_PLACEMENT_3D('',#22119,#18196,#18197);
#15767=AXIS2_PLACEMENT_3D('',#22121,#18199,#18200);
#15768=AXIS2_PLACEMENT_3D('',#22125,#18202,#18203);
#15769=AXIS2_PLACEMENT_3D('',#22129,#18205,#18206);
#15770=AXIS2_PLACEMENT_3D('',#22131,#18207,#18208);
#15771=AXIS2_PLACEMENT_3D('',#22133,#18209,#18210);
#15772=AXIS2_PLACEMENT_3D('',#22137,#18212,#18213);
#15773=AXIS2_PLACEMENT_3D('',#22141,#18215,#18216);
#15774=AXIS2_PLACEMENT_3D('',#22143,#18217,#18218);
#15775=AXIS2_PLACEMENT_3D('',#22145,#18219,#18220);
#15776=AXIS2_PLACEMENT_3D('',#22148,#18222,#18223);
#15777=AXIS2_PLACEMENT_3D('',#22149,#18224,#18225);
#15778=AXIS2_PLACEMENT_3D('',#22151,#18227,#18228);
#15779=AXIS2_PLACEMENT_3D('',#22153,#18230,#18231);
#15780=AXIS2_PLACEMENT_3D('',#22155,#18233,#18234);
#15781=AXIS2_PLACEMENT_3D('',#22157,#18236,#18237);
#15782=AXIS2_PLACEMENT_3D('',#22159,#18239,#18240);
#15783=AXIS2_PLACEMENT_3D('',#22161,#18242,#18243);
#15784=AXIS2_PLACEMENT_3D('',#22163,#18245,#18246);
#15785=AXIS2_PLACEMENT_3D('',#22165,#18248,#18249);
#15786=AXIS2_PLACEMENT_3D('',#22172,#18256,#18257);
#15787=AXIS2_PLACEMENT_3D('',#22174,#18259,#18260);
#15788=AXIS2_PLACEMENT_3D('',#22176,#18262,#18263);
#15789=AXIS2_PLACEMENT_3D('',#22178,#18265,#18266);
#15790=AXIS2_PLACEMENT_3D('',#22180,#18268,#18269);
#15791=AXIS2_PLACEMENT_3D('',#22182,#18271,#18272);
#15792=AXIS2_PLACEMENT_3D('',#22184,#18274,#18275);
#15793=AXIS2_PLACEMENT_3D('',#22186,#18277,#18278);
#15794=AXIS2_PLACEMENT_3D('',#22188,#18280,#18281);
#15795=AXIS2_PLACEMENT_3D('',#22190,#18283,#18284);
#15796=AXIS2_PLACEMENT_3D('',#22192,#18286,#18287);
#15797=AXIS2_PLACEMENT_3D('',#22194,#18289,#18290);
#15798=AXIS2_PLACEMENT_3D('',#22196,#18292,#18293);
#15799=AXIS2_PLACEMENT_3D('',#22202,#18297,#18298);
#15800=AXIS2_PLACEMENT_3D('',#22206,#18301,#18302);
#15801=AXIS2_PLACEMENT_3D('',#22212,#18306,#18307);
#15802=AXIS2_PLACEMENT_3D('',#22216,#18310,#18311);
#15803=AXIS2_PLACEMENT_3D('',#22220,#18314,#18315);
#15804=AXIS2_PLACEMENT_3D('',#22224,#18318,#18319);
#15805=AXIS2_PLACEMENT_3D('',#22226,#18321,#18322);
#15806=AXIS2_PLACEMENT_3D('',#22228,#18324,#18325);
#15807=AXIS2_PLACEMENT_3D('',#22231,#18328,#18329);
#15808=AXIS2_PLACEMENT_3D('',#22233,#18331,#18332);
#15809=AXIS2_PLACEMENT_3D('',#22235,#18334,#18335);
#15810=AXIS2_PLACEMENT_3D('',#22236,#18336,#18337);
#15811=AXIS2_PLACEMENT_3D('',#22239,#18340,#18341);
#15812=AXIS2_PLACEMENT_3D('',#22240,#18342,#18343);
#15813=AXIS2_PLACEMENT_3D('',#22241,#18344,#18345);
#15814=AXIS2_PLACEMENT_3D('',#22243,#18347,#18348);
#15815=AXIS2_PLACEMENT_3D('',#22245,#18350,#18351);
#18014=DIRECTION('axis',(0.,0.,1.));
#18015=DIRECTION('refdir',(1.,0.,0.));
#18016=DIRECTION('center_axis',(1.,0.,0.));
#18017=DIRECTION('ref_axis',(0.,0.,-1.));
#18018=DIRECTION('center_axis',(-1.,0.,0.));
#18019=DIRECTION('ref_axis',(0.,0.,-1.));
#18020=DIRECTION('',(0.70710678118654,-8.65956056235502E-17,0.707106781186555));
#18021=DIRECTION('center_axis',(1.,0.,0.));
#18022=DIRECTION('ref_axis',(0.,0.,-1.));
#18023=DIRECTION('center_axis',(1.,0.,0.));
#18024=DIRECTION('ref_axis',(0.,0.,-1.));
#18025=DIRECTION('center_axis',(1.,0.,0.));
#18026=DIRECTION('ref_axis',(0.,0.,-1.));
#18027=DIRECTION('',(0.,0.,1.));
#18028=DIRECTION('',(0.,-0.707106781186549,0.707106781186546));
#18029=DIRECTION('',(0.,1.,0.));
#18030=DIRECTION('',(0.,-0.923879532511287,-0.38268343236509));
#18031=DIRECTION('',(0.,0.707106781186547,0.707106781186548));
#18032=DIRECTION('',(0.,0.,1.));
#18033=DIRECTION('',(0.,1.,0.));
#18034=DIRECTION('',(0.,0.,-1.));
#18035=DIRECTION('',(0.,0.707106781186547,-0.707106781186548));
#18036=DIRECTION('',(0.,-0.923879532511287,0.38268343236509));
#18037=DIRECTION('',(0.,1.,0.));
#18038=DIRECTION('',(0.,1.,0.));
#18039=DIRECTION('',(0.,-0.707106781186547,-0.707106781186547));
#18040=DIRECTION('',(0.,0.,-1.));
#18041=DIRECTION('',(0.,0.707106781186547,-0.707106781186547));
#18042=DIRECTION('',(0.,-1.,0.));
#18043=DIRECTION('',(0.,0.70710678118655,0.707106781186545));
#18044=DIRECTION('center_axis',(-1.,0.,0.));
#18045=DIRECTION('ref_axis',(0.,0.,-1.));
#18046=DIRECTION('',(-1.,0.,0.));
#18047=DIRECTION('center_axis',(-1.,0.,0.));
#18048=DIRECTION('ref_axis',(0.,0.,-1.));
#18049=DIRECTION('center_axis',(-1.,0.,0.));
#18050=DIRECTION('ref_axis',(0.,0.,-1.));
#18051=DIRECTION('center_axis',(1.,0.,0.));
#18052=DIRECTION('ref_axis',(0.,1.,0.));
#18053=DIRECTION('',(0.515038074910058,-0.85716730070211,-1.04972719113862E-16));
#18054=DIRECTION('center_axis',(-1.,0.,0.));
#18055=DIRECTION('ref_axis',(0.,0.,-1.));
#18056=DIRECTION('center_axis',(1.,0.,0.));
#18057=DIRECTION('ref_axis',(0.,0.,-1.));
#18058=DIRECTION('',(-0.707106781186548,8.65956056235493E-17,0.707106781186547));
#18059=DIRECTION('center_axis',(-1.,0.,0.));
#18060=DIRECTION('ref_axis',(0.,0.,-1.));
#18061=DIRECTION('center_axis',(-1.,0.,0.));
#18062=DIRECTION('ref_axis',(0.,0.,-1.));
#18063=DIRECTION('center_axis',(1.,0.,0.));
#18064=DIRECTION('ref_axis',(0.,0.,-1.));
#18065=DIRECTION('',(0.,0.,1.));
#18066=DIRECTION('',(0.,0.707106781186547,0.707106781186547));
#18067=DIRECTION('',(0.,1.,0.));
#18068=DIRECTION('',(0.,1.,0.));
#18069=DIRECTION('',(0.,0.923879532511287,-0.38268343236509));
#18070=DIRECTION('',(0.,0.707106781186547,-0.707106781186548));
#18071=DIRECTION('',(0.,0.,-1.));
#18072=DIRECTION('',(0.,1.,0.));
#18073=DIRECTION('',(0.,0.,1.));
#18074=DIRECTION('',(0.,0.707106781186547,0.707106781186548));
#18075=DIRECTION('',(0.,0.923879532511287,0.38268343236509));
#18076=DIRECTION('',(0.,1.,0.));
#18077=DIRECTION('',(0.,0.707106781186549,-0.707106781186546));
#18078=DIRECTION('',(0.,0.,-1.));
#18079=DIRECTION('',(0.,-0.70710678118655,-0.707106781186545));
#18080=DIRECTION('',(0.,-1.,0.));
#18081=DIRECTION('',(0.,-0.707106781186547,0.707106781186547));
#18082=DIRECTION('center_axis',(1.,0.,0.));
#18083=DIRECTION('ref_axis',(0.,0.,-1.));
#18084=DIRECTION('',(1.,0.,0.));
#18085=DIRECTION('center_axis',(1.,0.,0.));
#18086=DIRECTION('ref_axis',(0.,0.,-1.));
#18087=DIRECTION('center_axis',(1.,0.,0.));
#18088=DIRECTION('ref_axis',(0.,0.,-1.));
#18089=DIRECTION('center_axis',(-1.,0.,0.));
#18090=DIRECTION('ref_axis',(0.,1.,0.));
#18091=DIRECTION('',(-0.515038074910058,-0.85716730070211,1.04972719113862E-16));
#18092=DIRECTION('center_axis',(0.,0.,1.));
#18093=DIRECTION('ref_axis',(1.,0.,0.));
#18094=DIRECTION('center_axis',(0.,0.,-1.));
#18095=DIRECTION('ref_axis',(1.,0.,0.));
#18096=DIRECTION('',(-0.707106781186564,-8.65956056235513E-17,0.707106781186531));
#18097=DIRECTION('center_axis',(0.,0.,1.));
#18098=DIRECTION('ref_axis',(1.,0.,0.));
#18099=DIRECTION('center_axis',(0.,0.,1.));
#18100=DIRECTION('ref_axis',(0.,-1.,0.));
#18101=DIRECTION('',(-1.,0.,0.));
#18102=DIRECTION('',(1.,0.,0.));
#18103=DIRECTION('center_axis',(0.,0.,1.));
#18104=DIRECTION('ref_axis',(1.,0.,0.));
#18105=DIRECTION('center_axis',(0.,0.,1.));
#18106=DIRECTION('ref_axis',(1.,0.,0.));
#18107=DIRECTION('center_axis',(0.,0.,1.));
#18108=DIRECTION('ref_axis',(1.,0.,0.));
#18109=DIRECTION('center_axis',(0.,0.,-1.));
#18110=DIRECTION('ref_axis',(1.,0.,0.));
#18111=DIRECTION('',(0.,0.,-1.));
#18112=DIRECTION('center_axis',(0.,0.,1.));
#18113=DIRECTION('ref_axis',(1.,0.,0.));
#18114=DIRECTION('',(0.,0.,1.));
#18115=DIRECTION('center_axis',(0.,0.707106781186548,0.707106781186547));
#18116=DIRECTION('ref_axis',(0.,-0.707106781186547,0.707106781186548));
#18117=DIRECTION('center_axis',(0.,0.,-1.));
#18118=DIRECTION('ref_axis',(1.,0.,0.));
#18119=DIRECTION('center_axis',(0.,0.707106781186548,0.707106781186547));
#18120=DIRECTION('ref_axis',(0.,-0.707106781186547,0.707106781186548));
#18121=DIRECTION('',(0.,0.,-1.));
#18122=DIRECTION('center_axis',(0.,0.,1.));
#18123=DIRECTION('ref_axis',(1.,0.,0.));
#18124=DIRECTION('',(0.,0.,1.));
#18125=DIRECTION('center_axis',(0.,-0.707106781186548,0.707106781186547));
#18126=DIRECTION('ref_axis',(0.,-0.707106781186547,-0.707106781186548));
#18127=DIRECTION('center_axis',(0.,0.,-1.));
#18128=DIRECTION('ref_axis',(1.,0.,0.));
#18129=DIRECTION('center_axis',(0.,-0.707106781186548,0.707106781186547));
#18130=DIRECTION('ref_axis',(0.,-0.707106781186547,-0.707106781186548));
#18131=DIRECTION('',(0.,0.,-1.));
#18132=DIRECTION('center_axis',(0.,0.,1.));
#18133=DIRECTION('ref_axis',(1.,0.,0.));
#18134=DIRECTION('center_axis',(0.,0.,1.));
#18135=DIRECTION('ref_axis',(1.,0.,0.));
#18136=DIRECTION('center_axis',(0.,0.,-1.));
#18137=DIRECTION('ref_axis',(1.,0.,0.));
#18138=DIRECTION('',(-0.707106781186547,-8.65956056235493E-17,0.707106781186548));
#18139=DIRECTION('center_axis',(0.,0.,-1.));
#18140=DIRECTION('ref_axis',(1.,0.,0.));
#18141=DIRECTION('',(0.,0.,-1.));
#18142=DIRECTION('center_axis',(0.,0.,1.));
#18143=DIRECTION('ref_axis',(1.,0.,0.));
#18144=DIRECTION('',(0.,0.,1.));
#18145=DIRECTION('center_axis',(0.,0.707106781186548,0.707106781186547));
#18146=DIRECTION('ref_axis',(0.,-0.707106781186547,0.707106781186548));
#18147=DIRECTION('center_axis',(0.,0.,-1.));
#18148=DIRECTION('ref_axis',(1.,0.,0.));
#18149=DIRECTION('center_axis',(0.,0.707106781186548,0.707106781186547));
#18150=DIRECTION('ref_axis',(0.,-0.707106781186547,0.707106781186548));
#18151=DIRECTION('',(0.,0.,-1.));
#18152=DIRECTION('center_axis',(0.,0.,1.));
#18153=DIRECTION('ref_axis',(1.,0.,0.));
#18154=DIRECTION('',(0.,0.,1.));
#18155=DIRECTION('center_axis',(0.,-0.707106781186548,0.707106781186547));
#18156=DIRECTION('ref_axis',(0.,-0.707106781186547,-0.707106781186548));
#18157=DIRECTION('center_axis',(0.,0.,-1.));
#18158=DIRECTION('ref_axis',(1.,0.,0.));
#18159=DIRECTION('center_axis',(0.,-0.707106781186548,0.707106781186547));
#18160=DIRECTION('ref_axis',(0.,-0.707106781186547,-0.707106781186548));
#18161=DIRECTION('',(0.,0.,-1.));
#18162=DIRECTION('center_axis',(0.,0.,1.));
#18163=DIRECTION('ref_axis',(1.,0.,0.));
#18164=DIRECTION('center_axis',(0.,0.,1.));
#18165=DIRECTION('ref_axis',(1.,0.,0.));
#18166=DIRECTION('center_axis',(0.,0.,-1.));
#18167=DIRECTION('ref_axis',(1.,0.,0.));
#18168=DIRECTION('',(-0.707106781186542,-8.65956056235487E-17,0.707106781186553));
#18169=DIRECTION('center_axis',(0.,0.,-1.));
#18170=DIRECTION('ref_axis',(1.,0.,0.));
#18171=DIRECTION('',(0.,0.,-1.));
#18172=DIRECTION('center_axis',(0.,0.,1.));
#18173=DIRECTION('ref_axis',(1.,0.,0.));
#18174=DIRECTION('',(0.,0.,1.));
#18175=DIRECTION('center_axis',(0.,0.707106781186548,0.707106781186547));
#18176=DIRECTION('ref_axis',(0.,-0.707106781186547,0.707106781186548));
#18177=DIRECTION('center_axis',(0.,0.,-1.));
#18178=DIRECTION('ref_axis',(1.,0.,0.));
#18179=DIRECTION('center_axis',(0.,0.707106781186548,0.707106781186547));
#18180=DIRECTION('ref_axis',(0.,-0.707106781186547,0.707106781186548));
#18181=DIRECTION('',(0.,0.,-1.));
#18182=DIRECTION('center_axis',(0.,0.,1.));
#18183=DIRECTION('ref_axis',(1.,0.,0.));
#18184=DIRECTION('',(0.,0.,1.));
#18185=DIRECTION('center_axis',(0.,-0.707106781186548,0.707106781186547));
#18186=DIRECTION('ref_axis',(0.,-0.707106781186547,-0.707106781186548));
#18187=DIRECTION('center_axis',(0.,0.,-1.));
#18188=DIRECTION('ref_axis',(1.,0.,0.));
#18189=DIRECTION('center_axis',(0.,-0.707106781186548,0.707106781186547));
#18190=DIRECTION('ref_axis',(0.,-0.707106781186547,-0.707106781186548));
#18191=DIRECTION('',(0.,0.,-1.));
#18192=DIRECTION('center_axis',(0.,0.,1.));
#18193=DIRECTION('ref_axis',(1.,0.,0.));
#18194=DIRECTION('center_axis',(0.,0.,1.));
#18195=DIRECTION('ref_axis',(1.,0.,0.));
#18196=DIRECTION('center_axis',(0.,0.,-1.));
#18197=DIRECTION('ref_axis',(1.,0.,0.));
#18198=DIRECTION('',(-0.707106781186542,-8.65956056235487E-17,0.707106781186553));
#18199=DIRECTION('center_axis',(0.,0.,-1.));
#18200=DIRECTION('ref_axis',(1.,0.,0.));
#18201=DIRECTION('',(0.,0.,-1.));
#18202=DIRECTION('center_axis',(0.,0.,1.));
#18203=DIRECTION('ref_axis',(1.,0.,0.));
#18204=DIRECTION('',(0.,0.,1.));
#18205=DIRECTION('center_axis',(0.,0.707106781186548,0.707106781186547));
#18206=DIRECTION('ref_axis',(0.,-0.707106781186547,0.707106781186548));
#18207=DIRECTION('center_axis',(0.,0.,-1.));
#18208=DIRECTION('ref_axis',(1.,0.,0.));
#18209=DIRECTION('center_axis',(0.,0.707106781186548,0.707106781186547));
#18210=DIRECTION('ref_axis',(0.,-0.707106781186547,0.707106781186548));
#18211=DIRECTION('',(0.,0.,-1.));
#18212=DIRECTION('center_axis',(0.,0.,1.));
#18213=DIRECTION('ref_axis',(1.,0.,0.));
#18214=DIRECTION('',(0.,0.,1.));
#18215=DIRECTION('center_axis',(0.,-0.707106781186548,0.707106781186547));
#18216=DIRECTION('ref_axis',(0.,-0.707106781186547,-0.707106781186548));
#18217=DIRECTION('center_axis',(0.,0.,-1.));
#18218=DIRECTION('ref_axis',(1.,0.,0.));
#18219=DIRECTION('center_axis',(0.,-0.707106781186548,0.707106781186547));
#18220=DIRECTION('ref_axis',(0.,-0.707106781186547,-0.707106781186548));
#18221=DIRECTION('',(0.,0.,-1.));
#18222=DIRECTION('center_axis',(0.,0.,1.));
#18223=DIRECTION('ref_axis',(1.,0.,0.));
#18224=DIRECTION('center_axis',(0.,0.,1.));
#18225=DIRECTION('ref_axis',(1.,0.,0.));
#18226=DIRECTION('',(-1.,0.,0.));
#18227=DIRECTION('center_axis',(0.,0.,1.));
#18228=DIRECTION('ref_axis',(1.,0.,0.));
#18229=DIRECTION('',(1.,0.,0.));
#18230=DIRECTION('center_axis',(0.,0.,1.));
#18231=DIRECTION('ref_axis',(1.,0.,0.));
#18232=DIRECTION('',(-1.,0.,0.));
#18233=DIRECTION('center_axis',(0.,0.,1.));
#18234=DIRECTION('ref_axis',(1.,0.,0.));
#18235=DIRECTION('',(1.,0.,0.));
#18236=DIRECTION('center_axis',(0.,0.,1.));
#18237=DIRECTION('ref_axis',(1.,0.,0.));
#18238=DIRECTION('',(-1.,0.,0.));
#18239=DIRECTION('center_axis',(0.,0.,1.));
#18240=DIRECTION('ref_axis',(1.,0.,0.));
#18241=DIRECTION('',(1.,0.,0.));
#18242=DIRECTION('center_axis',(0.,0.,1.));
#18243=DIRECTION('ref_axis',(1.,0.,0.));
#18244=DIRECTION('',(-1.,0.,0.));
#18245=DIRECTION('center_axis',(0.,0.,1.));
#18246=DIRECTION('ref_axis',(1.,0.,0.));
#18247=DIRECTION('',(1.,0.,0.));
#18248=DIRECTION('center_axis',(0.,0.707106781186548,-0.707106781186547));
#18249=DIRECTION('ref_axis',(0.,0.707106781186547,0.707106781186548));
#18250=DIRECTION('',(1.,0.,0.));
#18251=DIRECTION('',(1.,0.,0.));
#18252=DIRECTION('',(1.,0.,0.));
#18253=DIRECTION('',(1.,0.,0.));
#18254=DIRECTION('',(1.,0.,0.));
#18255=DIRECTION('',(1.,0.,0.));
#18256=DIRECTION('center_axis',(0.,1.,0.));
#18257=DIRECTION('ref_axis',(0.,0.,1.));
#18258=DIRECTION('',(1.,0.,0.));
#18259=DIRECTION('center_axis',(0.,1.,0.));
#18260=DIRECTION('ref_axis',(0.,0.,1.));
#18261=DIRECTION('',(1.,0.,0.));
#18262=DIRECTION('center_axis',(0.,1.,0.));
#18263=DIRECTION('ref_axis',(0.,0.,1.));
#18264=DIRECTION('',(1.,0.,0.));
#18265=DIRECTION('center_axis',(0.,1.,0.));
#18266=DIRECTION('ref_axis',(0.,0.,1.));
#18267=DIRECTION('',(1.,0.,0.));
#18268=DIRECTION('center_axis',(0.,0.,-1.));
#18269=DIRECTION('ref_axis',(0.,1.,0.));
#18270=DIRECTION('',(1.,0.,0.));
#18271=DIRECTION('center_axis',(0.,0.,-1.));
#18272=DIRECTION('ref_axis',(0.,1.,0.));
#18273=DIRECTION('',(1.,0.,0.));
#18274=DIRECTION('center_axis',(0.,0.,-1.));
#18275=DIRECTION('ref_axis',(0.,1.,0.));
#18276=DIRECTION('',(1.,0.,0.));
#18277=DIRECTION('center_axis',(0.,0.,-1.));
#18278=DIRECTION('ref_axis',(0.,1.,0.));
#18279=DIRECTION('',(1.,0.,0.));
#18280=DIRECTION('center_axis',(0.,-1.,0.));
#18281=DIRECTION('ref_axis',(0.,0.,-1.));
#18282=DIRECTION('',(1.,0.,0.));
#18283=DIRECTION('center_axis',(0.,-1.,0.));
#18284=DIRECTION('ref_axis',(0.,0.,-1.));
#18285=DIRECTION('',(1.,0.,0.));
#18286=DIRECTION('center_axis',(0.,-1.,0.));
#18287=DIRECTION('ref_axis',(0.,0.,-1.));
#18288=DIRECTION('',(1.,0.,0.));
#18289=DIRECTION('center_axis',(0.,-1.,0.));
#18290=DIRECTION('ref_axis',(0.,0.,-1.));
#18291=DIRECTION('',(1.,0.,0.));
#18292=DIRECTION('center_axis',(0.707106781186534,-0.707106781186561,0.));
#18293=DIRECTION('ref_axis',(0.,0.,-1.));
#18294=DIRECTION('',(0.577350269189641,0.57735026918962,-0.577350269189617));
#18295=DIRECTION('',(-0.577350269189641,-0.57735026918962,-0.577350269189616));
#18296=DIRECTION('',(0.,0.,-1.));
#18297=DIRECTION('center_axis',(0.,-0.707106781186545,0.70710678118655));
#18298=DIRECTION('ref_axis',(1.,0.,0.));
#18299=DIRECTION('',(-0.577350269189628,0.577350269189626,0.577350269189623));
#18300=DIRECTION('',(1.,0.,0.));
#18301=DIRECTION('center_axis',(0.707106781186532,0.707106781186563,0.));
#18302=DIRECTION('ref_axis',(0.,0.,-1.));
#18303=DIRECTION('',(0.577350269189643,-0.577350269189617,0.577350269189617));
#18304=DIRECTION('',(-0.577350269189643,0.577350269189617,0.577350269189617));
#18305=DIRECTION('',(0.,0.,1.));
#18306=DIRECTION('center_axis',(0.,0.707106781186548,0.707106781186548));
#18307=DIRECTION('ref_axis',(1.,0.,0.));
#18308=DIRECTION('',(-1.,0.,0.));
#18309=DIRECTION('',(0.577350269189629,0.577350269189624,-0.577350269189624));
#18310=DIRECTION('center_axis',(-0.707106781186545,0.70710678118655,0.));
#18311=DIRECTION('ref_axis',(0.,0.,1.));
#18312=DIRECTION('',(0.,0.,-1.));
#18313=DIRECTION('',(-0.577350269189629,-0.577350269189624,-0.577350269189624));
#18314=DIRECTION('center_axis',(-0.707106781186546,-0.707106781186549,0.));
#18315=DIRECTION('ref_axis',(0.,0.,1.));
#18316=DIRECTION('',(0.577350269189628,-0.577350269189626,0.577350269189623));
#18317=DIRECTION('',(0.,0.,1.));
#18318=DIRECTION('center_axis',(0.,0.38268343236509,-0.923879532511287));
#18319=DIRECTION('ref_axis',(-1.,0.,0.));
#18320=DIRECTION('',(-1.,0.,0.));
#18321=DIRECTION('center_axis',(0.,0.,-1.));
#18322=DIRECTION('ref_axis',(0.,1.,0.));
#18323=DIRECTION('',(1.,0.,0.));
#18324=DIRECTION('center_axis',(0.,-0.38268343236509,-0.923879532511287));
#18325=DIRECTION('ref_axis',(-1.,0.,0.));
#18326=DIRECTION('',(-1.,0.,0.));
#18327=DIRECTION('',(1.,0.,0.));
#18328=DIRECTION('center_axis',(0.,-0.707106781186548,-0.707106781186547));
#18329=DIRECTION('ref_axis',(0.,0.707106781186547,-0.707106781186548));
#18330=DIRECTION('',(1.,0.,0.));
#18331=DIRECTION('center_axis',(0.,-1.,0.));
#18332=DIRECTION('ref_axis',(0.,0.,-1.));
#18333=DIRECTION('',(-1.,0.,0.));
#18334=DIRECTION('center_axis',(0.,-0.707106781186546,-0.707106781186549));
#18335=DIRECTION('ref_axis',(-1.,0.,0.));
#18336=DIRECTION('center_axis',(0.,0.707106781186548,-0.707106781186548));
#18337=DIRECTION('ref_axis',(-1.,0.,0.));
#18338=DIRECTION('',(-1.,0.,0.));
#18339=DIRECTION('',(1.,0.,0.));
#18340=DIRECTION('center_axis',(0.,0.,-1.));
#18341=DIRECTION('ref_axis',(0.,1.,0.));
#18342=DIRECTION('center_axis',(0.,1.,0.));
#18343=DIRECTION('ref_axis',(0.,0.,1.));
#18344=DIRECTION('center_axis',(0.,-1.,0.));
#18345=DIRECTION('ref_axis',(0.,0.,-1.));
#18346=DIRECTION('',(1.,0.,0.));
#18347=DIRECTION('center_axis',(0.,0.,-1.));
#18348=DIRECTION('ref_axis',(0.,1.,0.));
#18349=DIRECTION('',(1.,0.,0.));
#18350=DIRECTION('center_axis',(0.,1.,0.));
#18351=DIRECTION('ref_axis',(0.,0.,1.));
#21907=CARTESIAN_POINT('',(0.,0.,0.));
#21908=CARTESIAN_POINT('Origin',(204.9,31.,34.5));
#21909=CARTESIAN_POINT('',(204.8,31.,36.05));
#21910=CARTESIAN_POINT('Origin',(204.8,31.,34.5));
#21911=CARTESIAN_POINT('',(205.,31.,36.25));
#21912=CARTESIAN_POINT('',(204.9,31.,36.15));
#21913=CARTESIAN_POINT('',(205.,31.,32.75));
#21914=CARTESIAN_POINT('Origin',(205.,31.,34.5));
#21915=CARTESIAN_POINT('Origin',(205.,31.,34.5));
#21916=CARTESIAN_POINT('Origin',(205.,21.,36.125));
#21917=CARTESIAN_POINT('',(205.,6.3,32.95));
#21918=CARTESIAN_POINT('',(205.,6.3,39.3));
#21919=CARTESIAN_POINT('',(205.,6.3,37.8125));
#21920=CARTESIAN_POINT('',(205.,6.5,32.75));
#21921=CARTESIAN_POINT('',(205.,9.15625000000002,30.09375));
#21922=CARTESIAN_POINT('',(205.,17.304,32.75));
#21923=CARTESIAN_POINT('',(205.,6.,32.75));
#21924=CARTESIAN_POINT('',(205.,17.6454213562373,32.8914213562373));
#21925=CARTESIAN_POINT('',(205.,19.5633433515018,33.6858506582495));
#21926=CARTESIAN_POINT('',(205.,20.4,35.646));
#21927=CARTESIAN_POINT('',(205.,17.504,32.75));
#21928=CARTESIAN_POINT('',(205.,20.4,36.846));
#21929=CARTESIAN_POINT('',(205.,20.4,35.646));
#21930=CARTESIAN_POINT('',(205.,21.6,36.846));
#21931=CARTESIAN_POINT('',(205.,20.4,36.846));
#21932=CARTESIAN_POINT('',(205.,21.6,35.646));
#21933=CARTESIAN_POINT('',(205.,21.6,36.846));
#21934=CARTESIAN_POINT('',(205.,24.3545786437627,32.8914213562373));
#21935=CARTESIAN_POINT('',(205.,21.6,35.646));
#21936=CARTESIAN_POINT('',(205.,24.696,32.75));
#21937=CARTESIAN_POINT('',(205.,22.4366566484982,33.6858506582495));
#21938=CARTESIAN_POINT('',(205.,24.496,32.75));
#21939=CARTESIAN_POINT('',(205.,35.5,32.75));
#21940=CARTESIAN_POINT('',(205.,24.496,32.75));
#21941=CARTESIAN_POINT('',(205.,35.7,32.95));
#21942=CARTESIAN_POINT('',(205.,32.84375,30.09375));
#21943=CARTESIAN_POINT('',(205.,35.7,39.3));
#21944=CARTESIAN_POINT('',(205.,35.7,34.4375));
#21945=CARTESIAN_POINT('',(205.,35.5,39.5));
#21946=CARTESIAN_POINT('',(205.,32.84375,42.15625));
#21947=CARTESIAN_POINT('',(205.,6.5,39.5));
#21948=CARTESIAN_POINT('',(205.,36.,39.5));
#21949=CARTESIAN_POINT('',(205.,9.15625000000002,42.15625));
#21950=CARTESIAN_POINT('Origin',(205.,31.,34.5));
#21951=CARTESIAN_POINT('',(198.,31.,36.05));
#21952=CARTESIAN_POINT('',(205.,31.,36.05));
#21953=CARTESIAN_POINT('',(198.,29.45,34.5));
#21954=CARTESIAN_POINT('Origin',(198.,31.,34.5));
#21955=CARTESIAN_POINT('Origin',(198.,31.,34.5));
#21956=CARTESIAN_POINT('Origin',(197.534333020254,31.,34.5));
#21957=CARTESIAN_POINT('',(197.068666040507,31.,34.5));
#21958=CARTESIAN_POINT('',(197.534333020254,30.225,34.5));
#21959=CARTESIAN_POINT('Origin',(5.1,31.,34.5));
#21960=CARTESIAN_POINT('',(5.2,31.,36.05));
#21961=CARTESIAN_POINT('Origin',(5.2,31.,34.5));
#21962=CARTESIAN_POINT('',(5.,31.,36.25));
#21963=CARTESIAN_POINT('',(5.1,31.,36.15));
#21964=CARTESIAN_POINT('',(5.,31.,32.75));
#21965=CARTESIAN_POINT('Origin',(5.,31.,34.5));
#21966=CARTESIAN_POINT('Origin',(5.,31.,34.5));
#21967=CARTESIAN_POINT('Origin',(5.,21.,36.125));
#21968=CARTESIAN_POINT('',(5.,35.7,32.95));
#21969=CARTESIAN_POINT('',(5.,35.7,39.3));
#21970=CARTESIAN_POINT('',(5.,35.7,34.4375));
#21971=CARTESIAN_POINT('',(5.,35.5,32.75));
#21972=CARTESIAN_POINT('',(5.,32.84375,30.09375));
#21973=CARTESIAN_POINT('',(5.,24.496,32.75));
#21974=CARTESIAN_POINT('',(5.,24.696,32.75));
#21975=CARTESIAN_POINT('',(5.,24.496,32.75));
#21976=CARTESIAN_POINT('',(5.,24.3545786437627,32.8914213562373));
#21977=CARTESIAN_POINT('',(5.,22.4366566484982,33.6858506582495));
#21978=CARTESIAN_POINT('',(5.,21.6,35.646));
#21979=CARTESIAN_POINT('',(5.,21.6,35.646));
#21980=CARTESIAN_POINT('',(5.,21.6,36.846));
#21981=CARTESIAN_POINT('',(5.,21.6,36.846));
#21982=CARTESIAN_POINT('',(5.,20.4,36.846));
#21983=CARTESIAN_POINT('',(5.,20.4,36.846));
#21984=CARTESIAN_POINT('',(5.,20.4,35.646));
#21985=CARTESIAN_POINT('',(5.,20.4,35.646));
#21986=CARTESIAN_POINT('',(5.,17.6454213562373,32.8914213562373));
#21987=CARTESIAN_POINT('',(5.,17.504,32.75));
#21988=CARTESIAN_POINT('',(5.,17.304,32.75));
#21989=CARTESIAN_POINT('',(5.,19.5633433515018,33.6858506582495));
#21990=CARTESIAN_POINT('',(5.,6.5,32.75));
#21991=CARTESIAN_POINT('',(5.,6.,32.75));
#21992=CARTESIAN_POINT('',(5.,6.3,32.95));
#21993=CARTESIAN_POINT('',(5.,9.15625000000002,30.09375));
#21994=CARTESIAN_POINT('',(5.,6.3,39.3));
#21995=CARTESIAN_POINT('',(5.,6.3,37.8125));
#21996=CARTESIAN_POINT('',(5.,6.5,39.5));
#21997=CARTESIAN_POINT('',(5.,9.15625000000002,42.15625));
#21998=CARTESIAN_POINT('',(5.,35.5,39.5));
#21999=CARTESIAN_POINT('',(5.,36.,39.5));
#22000=CARTESIAN_POINT('',(5.,32.84375,42.15625));
#22001=CARTESIAN_POINT('Origin',(5.,31.,34.5));
#22002=CARTESIAN_POINT('',(12.,31.,36.05));
#22003=CARTESIAN_POINT('',(5.,31.,36.05));
#22004=CARTESIAN_POINT('',(12.,29.45,34.5));
#22005=CARTESIAN_POINT('Origin',(12.,31.,34.5));
#22006=CARTESIAN_POINT('Origin',(12.,31.,34.5));
#22007=CARTESIAN_POINT('Origin',(12.,31.,34.5));
#22008=CARTESIAN_POINT('',(12.9313339594927,31.,34.5));
#22009=CARTESIAN_POINT('',(12.,29.45,34.5));
#22010=CARTESIAN_POINT('Origin',(180.,21.,39.35));
#22011=CARTESIAN_POINT('',(177.45,21.,39.2));
#22012=CARTESIAN_POINT('Origin',(180.,21.,39.2));
#22013=CARTESIAN_POINT('',(177.15,21.,39.5));
#22014=CARTESIAN_POINT('',(177.3,21.,39.35));
#22015=CARTESIAN_POINT('Origin',(180.,21.,39.5));
#22016=CARTESIAN_POINT('Origin',(5.,36.,39.5));
#22017=CARTESIAN_POINT('',(5.,6.5,39.5));
#22018=CARTESIAN_POINT('',(5.,35.5,39.5));
#22019=CARTESIAN_POINT('',(27.15,21.,39.5));
#22020=CARTESIAN_POINT('Origin',(30.,21.,39.5));
#22021=CARTESIAN_POINT('',(127.15,21.,39.5));
#22022=CARTESIAN_POINT('Origin',(130.,21.,39.5));
#22023=CARTESIAN_POINT('',(77.15,21.,39.5));
#22024=CARTESIAN_POINT('Origin',(80.,21.,39.5));
#22025=CARTESIAN_POINT('Origin',(180.,21.,39.5));
#22026=CARTESIAN_POINT('',(177.45,21.,36.846));
#22027=CARTESIAN_POINT('',(177.45,21.,39.5));
#22028=CARTESIAN_POINT('',(177.521593253721,21.6,36.846));
#22029=CARTESIAN_POINT('Origin',(180.,21.,36.846));
#22030=CARTESIAN_POINT('',(177.521593253721,21.6,35.646));
#22031=CARTESIAN_POINT('',(177.521593253721,21.6,39.5));
#22032=CARTESIAN_POINT('',(177.545690321088,21.692,35.554));
#22033=CARTESIAN_POINT('Origin',(180.,21.,36.246));
#22034=CARTESIAN_POINT('',(182.454309678912,21.692,35.554));
#22035=CARTESIAN_POINT('Origin',(180.,21.,35.554));
#22036=CARTESIAN_POINT('',(182.478406746279,21.6,35.646));
#22037=CARTESIAN_POINT('Origin',(180.,21.,36.246));
#22038=CARTESIAN_POINT('',(182.478406746279,21.6,36.846));
#22039=CARTESIAN_POINT('',(182.478406746279,21.6,39.5));
#22040=CARTESIAN_POINT('',(182.478406746279,20.4,36.846));
#22041=CARTESIAN_POINT('Origin',(180.,21.,36.846));
#22042=CARTESIAN_POINT('',(182.478406746279,20.4,35.646));
#22043=CARTESIAN_POINT('',(182.478406746279,20.4,39.5));
#22044=CARTESIAN_POINT('',(182.454309678912,20.308,35.554));
#22045=CARTESIAN_POINT('Origin',(180.,21.,36.246));
#22046=CARTESIAN_POINT('',(177.545690321088,20.308,35.554));
#22047=CARTESIAN_POINT('Origin',(180.,21.,35.554));
#22048=CARTESIAN_POINT('',(177.521593253721,20.4,35.646));
#22049=CARTESIAN_POINT('Origin',(180.,21.,36.246));
#22050=CARTESIAN_POINT('',(177.521593253721,20.4,36.846));
#22051=CARTESIAN_POINT('',(177.521593253721,20.4,39.5));
#22052=CARTESIAN_POINT('Origin',(180.,21.,36.846));
#22053=CARTESIAN_POINT('Origin',(30.,21.,39.35));
#22054=CARTESIAN_POINT('',(27.45,21.,39.2));
#22055=CARTESIAN_POINT('Origin',(30.,21.,39.2));
#22056=CARTESIAN_POINT('',(27.3,21.,39.35));
#22057=CARTESIAN_POINT('Origin',(30.,21.,39.5));
#22058=CARTESIAN_POINT('',(27.45,21.,36.846));
#22059=CARTESIAN_POINT('',(27.45,21.,39.5));
#22060=CARTESIAN_POINT('',(27.5215932537213,21.6,36.846));
#22061=CARTESIAN_POINT('Origin',(30.,21.,36.846));
#22062=CARTESIAN_POINT('',(27.5215932537213,21.6,35.646));
#22063=CARTESIAN_POINT('',(27.5215932537213,21.6,39.5));
#22064=CARTESIAN_POINT('',(27.5456903210882,21.692,35.554));
#22065=CARTESIAN_POINT('Origin',(30.,21.,36.246));
#22066=CARTESIAN_POINT('',(32.4543096789118,21.692,35.554));
#22067=CARTESIAN_POINT('Origin',(30.,21.,35.554));
#22068=CARTESIAN_POINT('',(32.4784067462787,21.6,35.646));
#22069=CARTESIAN_POINT('Origin',(30.,21.,36.246));
#22070=CARTESIAN_POINT('',(32.4784067462787,21.6,36.846));
#22071=CARTESIAN_POINT('',(32.4784067462787,21.6,39.5));
#22072=CARTESIAN_POINT('',(32.4784067462787,20.4,36.846));
#22073=CARTESIAN_POINT('Origin',(30.,21.,36.846));
#22074=CARTESIAN_POINT('',(32.4784067462787,20.4,35.646));
#22075=CARTESIAN_POINT('',(32.4784067462787,20.4,39.5));
#22076=CARTESIAN_POINT('',(32.4543096789118,20.308,35.554));
#22077=CARTESIAN_POINT('Origin',(30.,21.,36.246));
#22078=CARTESIAN_POINT('',(27.5456903210882,20.308,35.554));
#22079=CARTESIAN_POINT('Origin',(30.,21.,35.554));
#22080=CARTESIAN_POINT('',(27.5215932537213,20.4,35.646));
#22081=CARTESIAN_POINT('Origin',(30.,21.,36.246));
#22082=CARTESIAN_POINT('',(27.5215932537213,20.4,36.846));
#22083=CARTESIAN_POINT('',(27.5215932537213,20.4,39.5));
#22084=CARTESIAN_POINT('Origin',(30.,21.,36.846));
#22085=CARTESIAN_POINT('Origin',(80.,21.,39.35));
#22086=CARTESIAN_POINT('',(77.45,21.,39.2));
#22087=CARTESIAN_POINT('Origin',(80.,21.,39.2));
#22088=CARTESIAN_POINT('',(77.3,21.,39.35));
#22089=CARTESIAN_POINT('Origin',(80.,21.,39.5));
#22090=CARTESIAN_POINT('',(77.45,21.,36.846));
#22091=CARTESIAN_POINT('',(77.45,21.,39.5));
#22092=CARTESIAN_POINT('',(77.5215932537212,21.6,36.846));
#22093=CARTESIAN_POINT('Origin',(80.,21.,36.846));
#22094=CARTESIAN_POINT('',(77.5215932537212,21.6,35.646));
#22095=CARTESIAN_POINT('',(77.5215932537212,21.6,39.5));
#22096=CARTESIAN_POINT('',(77.5456903210882,21.692,35.554));
#22097=CARTESIAN_POINT('Origin',(80.,21.,36.246));
#22098=CARTESIAN_POINT('',(82.4543096789118,21.692,35.554));
#22099=CARTESIAN_POINT('Origin',(80.,21.,35.554));
#22100=CARTESIAN_POINT('',(82.4784067462788,21.6,35.646));
#22101=CARTESIAN_POINT('Origin',(80.,21.,36.246));
#22102=CARTESIAN_POINT('',(82.4784067462788,21.6,36.846));
#22103=CARTESIAN_POINT('',(82.4784067462788,21.6,39.5));
#22104=CARTESIAN_POINT('',(82.4784067462788,20.4,36.846));
#22105=CARTESIAN_POINT('Origin',(80.,21.,36.846));
#22106=CARTESIAN_POINT('',(82.4784067462788,20.4,35.646));
#22107=CARTESIAN_POINT('',(82.4784067462788,20.4,39.5));
#22108=CARTESIAN_POINT('',(82.4543096789118,20.308,35.554));
#22109=CARTESIAN_POINT('Origin',(80.,21.,36.246));
#22110=CARTESIAN_POINT('',(77.5456903210882,20.308,35.554));
#22111=CARTESIAN_POINT('Origin',(80.,21.,35.554));
#22112=CARTESIAN_POINT('',(77.5215932537212,20.4,35.646));
#22113=CARTESIAN_POINT('Origin',(80.,21.,36.246));
#22114=CARTESIAN_POINT('',(77.5215932537212,20.4,36.846));
#22115=CARTESIAN_POINT('',(77.5215932537212,20.4,39.5));
#22116=CARTESIAN_POINT('Origin',(80.,21.,36.846));
#22117=CARTESIAN_POINT('Origin',(130.,21.,39.35));
#22118=CARTESIAN_POINT('',(127.45,21.,39.2));
#22119=CARTESIAN_POINT('Origin',(130.,21.,39.2));
#22120=CARTESIAN_POINT('',(127.3,21.,39.35));
#22121=CARTESIAN_POINT('Origin',(130.,21.,39.5));
#22122=CARTESIAN_POINT('',(127.45,21.,36.846));
#22123=CARTESIAN_POINT('',(127.45,21.,39.5));
#22124=CARTESIAN_POINT('',(127.521593253721,21.6,36.846));
#22125=CARTESIAN_POINT('Origin',(130.,21.,36.846));
#22126=CARTESIAN_POINT('',(127.521593253721,21.6,35.646));
#22127=CARTESIAN_POINT('',(127.521593253721,21.6,39.5));
#22128=CARTESIAN_POINT('',(127.545690321088,21.692,35.554));
#22129=CARTESIAN_POINT('Origin',(130.,21.,36.246));
#22130=CARTESIAN_POINT('',(132.454309678912,21.692,35.554));
#22131=CARTESIAN_POINT('Origin',(130.,21.,35.554));
#22132=CARTESIAN_POINT('',(132.478406746279,21.6,35.646));
#22133=CARTESIAN_POINT('Origin',(130.,21.,36.246));
#22134=CARTESIAN_POINT('',(132.478406746279,21.6,36.846));
#22135=CARTESIAN_POINT('',(132.478406746279,21.6,39.5));
#22136=CARTESIAN_POINT('',(132.478406746279,20.4,36.846));
#22137=CARTESIAN_POINT('Origin',(130.,21.,36.846));
#22138=CARTESIAN_POINT('',(132.478406746279,20.4,35.646));
#22139=CARTESIAN_POINT('',(132.478406746279,20.4,39.5));
#22140=CARTESIAN_POINT('',(132.454309678912,20.308,35.554));
#22141=CARTESIAN_POINT('Origin',(130.,21.,36.246));
#22142=CARTESIAN_POINT('',(127.545690321088,20.308,35.554));
#22143=CARTESIAN_POINT('Origin',(130.,21.,35.554));
#22144=CARTESIAN_POINT('',(127.521593253721,20.4,35.646));
#22145=CARTESIAN_POINT('Origin',(130.,21.,36.246));
#22146=CARTESIAN_POINT('',(127.521593253721,20.4,36.846));
#22147=CARTESIAN_POINT('',(127.521593253721,20.4,39.5));
#22148=CARTESIAN_POINT('Origin',(130.,21.,36.846));
#22149=CARTESIAN_POINT('Origin',(130.,21.,35.554));
#22150=CARTESIAN_POINT('',(67.5,21.692,35.554));
#22151=CARTESIAN_POINT('Origin',(130.,21.,35.554));
#22152=CARTESIAN_POINT('',(67.5,20.308,35.554));
#22153=CARTESIAN_POINT('Origin',(80.,21.,35.554));
#22154=CARTESIAN_POINT('',(42.5,21.692,35.554));
#22155=CARTESIAN_POINT('Origin',(80.,21.,35.554));
#22156=CARTESIAN_POINT('',(42.5,20.308,35.554));
#22157=CARTESIAN_POINT('Origin',(30.,21.,35.554));
#22158=CARTESIAN_POINT('',(17.5,21.692,35.554));
#22159=CARTESIAN_POINT('Origin',(30.,21.,35.554));
#22160=CARTESIAN_POINT('',(17.5,20.308,35.554));
#22161=CARTESIAN_POINT('Origin',(180.,21.,35.554));
#22162=CARTESIAN_POINT('',(92.5,21.692,35.554));
#22163=CARTESIAN_POINT('Origin',(180.,21.,35.554));
#22164=CARTESIAN_POINT('',(92.5,20.308,35.554));
#22165=CARTESIAN_POINT('Origin',(5.,17.504,32.75));
#22166=CARTESIAN_POINT('',(5.,20.4,35.646));
#22167=CARTESIAN_POINT('',(5.,20.4,35.646));
#22168=CARTESIAN_POINT('',(5.,17.6454213562373,32.8914213562373));
#22169=CARTESIAN_POINT('',(5.,20.4,35.646));
#22170=CARTESIAN_POINT('',(5.,20.4,35.646));
#22171=CARTESIAN_POINT('',(5.,20.4,35.646));
#22172=CARTESIAN_POINT('Origin',(5.,20.4,35.646));
#22173=CARTESIAN_POINT('',(5.,20.4,36.846));
#22174=CARTESIAN_POINT('Origin',(5.,20.4,35.646));
#22175=CARTESIAN_POINT('',(5.,20.4,36.846));
#22176=CARTESIAN_POINT('Origin',(5.,20.4,35.646));
#22177=CARTESIAN_POINT('',(5.,20.4,36.846));
#22178=CARTESIAN_POINT('Origin',(5.,20.4,35.646));
#22179=CARTESIAN_POINT('',(5.,20.4,36.846));
#22180=CARTESIAN_POINT('Origin',(5.,20.4,36.846));
#22181=CARTESIAN_POINT('',(5.,21.6,36.846));
#22182=CARTESIAN_POINT('Origin',(5.,20.4,36.846));
#22183=CARTESIAN_POINT('',(5.,21.6,36.846));
#22184=CARTESIAN_POINT('Origin',(5.,20.4,36.846));
#22185=CARTESIAN_POINT('',(5.,21.6,36.846));
#22186=CARTESIAN_POINT('Origin',(5.,20.4,36.846));
#22187=CARTESIAN_POINT('',(5.,21.6,36.846));
#22188=CARTESIAN_POINT('Origin',(5.,21.6,36.846));
#22189=CARTESIAN_POINT('',(5.,21.6,35.646));
#22190=CARTESIAN_POINT('Origin',(5.,21.6,36.846));
#22191=CARTESIAN_POINT('',(5.,21.6,35.646));
#22192=CARTESIAN_POINT('Origin',(5.,21.6,36.846));
#22193=CARTESIAN_POINT('',(5.,21.6,35.646));
#22194=CARTESIAN_POINT('Origin',(5.,21.6,36.846));
#22195=CARTESIAN_POINT('',(5.,21.6,35.646));
#22196=CARTESIAN_POINT('Origin',(204.85,6.15,37.8125));
#22197=CARTESIAN_POINT('',(204.7,6.,33.25));
#22198=CARTESIAN_POINT('',(170.789583333332,-27.9104166666672,67.160416666667));
#22199=CARTESIAN_POINT('',(204.7,6.,39.));
#22200=CARTESIAN_POINT('',(171.352083333332,-27.3479166666672,5.652083333333));
#22201=CARTESIAN_POINT('',(204.7,6.,37.8125));
#22202=CARTESIAN_POINT('Origin',(5.,6.25,39.25));
#22203=CARTESIAN_POINT('',(5.3,6.,39.));
#22204=CARTESIAN_POINT('',(5.31458333333333,5.98541666666667,38.9854166666667));
#22205=CARTESIAN_POINT('',(5.,6.,39.));
#22206=CARTESIAN_POINT('Origin',(204.85,35.85,34.4375));
#22207=CARTESIAN_POINT('',(204.7,36.,39.));
#22208=CARTESIAN_POINT('',(170.789583333331,69.9104166666672,5.08958333333285));
#22209=CARTESIAN_POINT('',(204.7,36.,33.25));
#22210=CARTESIAN_POINT('',(171.352083333331,69.3479166666672,66.5979166666672));
#22211=CARTESIAN_POINT('',(204.7,36.,34.4375));
#22212=CARTESIAN_POINT('Origin',(5.,35.75,39.25));
#22213=CARTESIAN_POINT('',(5.3,36.,39.));
#22214=CARTESIAN_POINT('',(5.,36.,39.));
#22215=CARTESIAN_POINT('',(5.87708333333334,36.5770833333333,38.4229166666667));
#22216=CARTESIAN_POINT('Origin',(5.15,35.85,34.4375));
#22217=CARTESIAN_POINT('',(5.3,36.,33.25));
#22218=CARTESIAN_POINT('',(5.3,36.,34.4375));
#22219=CARTESIAN_POINT('',(5.31458333333333,36.0145833333333,33.2645833333333));
#22220=CARTESIAN_POINT('Origin',(5.15,6.15,37.8125));
#22221=CARTESIAN_POINT('',(5.3,6.,33.25));
#22222=CARTESIAN_POINT('',(5.87708333333333,5.42291666666667,33.8270833333333));
#22223=CARTESIAN_POINT('',(5.3,6.,37.8125));
#22224=CARTESIAN_POINT('Origin',(5.,17.4747106781187,32.8207106781187));
#22225=CARTESIAN_POINT('',(5.,17.304,32.75));
#22226=CARTESIAN_POINT('Origin',(5.,6.,32.75));
#22227=CARTESIAN_POINT('',(5.,6.5,32.75));
#22228=CARTESIAN_POINT('Origin',(5.,24.5252893218813,32.8207106781187));
#22229=CARTESIAN_POINT('',(5.,24.3545786437627,32.8914213562373));
#22230=CARTESIAN_POINT('',(5.,24.696,32.75));
#22231=CARTESIAN_POINT('Origin',(5.,21.6,35.646));
#22232=CARTESIAN_POINT('',(5.,21.6,35.646));
#22233=CARTESIAN_POINT('Origin',(5.,6.,39.5));
#22234=CARTESIAN_POINT('',(5.,6.,33.25));
#22235=CARTESIAN_POINT('Origin',(5.,6.25,33.));
#22236=CARTESIAN_POINT('Origin',(5.,35.75,33.));
#22237=CARTESIAN_POINT('',(5.,35.5,32.75));
#22238=CARTESIAN_POINT('',(5.,36.,33.25));
#22239=CARTESIAN_POINT('Origin',(5.,24.496,32.75));
#22240=CARTESIAN_POINT('Origin',(5.,36.,32.75));
#22241=CARTESIAN_POINT('Origin',(5.,21.6,36.846));
#22242=CARTESIAN_POINT('',(5.,21.6,36.846));
#22243=CARTESIAN_POINT('Origin',(5.,20.4,36.846));
#22244=CARTESIAN_POINT('',(5.,20.4,36.846));
#22245=CARTESIAN_POINT('Origin',(5.,20.4,35.646));
#81021=UNCERTAINTY_MEASURE_WITH_UNIT(LENGTH_MEASURE(0.01),#81041,
'DISTANCE_ACCURACY_VALUE',
'Maximum model space distance between geometric entities at asserted c
onnectivities');
#81028=UNCERTAINTY_MEASURE_WITH_UNIT(LENGTH_MEASURE(0.01),#81041,
'DISTANCE_ACCURACY_VALUE',
'Maximum model space distance between geometric entities at asserted c
onnectivities');
#81033=(
GEOMETRIC_REPRESENTATION_CONTEXT(3)
GLOBAL_UNCERTAINTY_ASSIGNED_CONTEXT((#81021))
GLOBAL_UNIT_ASSIGNED_CONTEXT((#81041,#81043,#81044))
REPRESENTATION_CONTEXT('','3D')
);
#81040=(
GEOMETRIC_REPRESENTATION_CONTEXT(3)
GLOBAL_UNCERTAINTY_ASSIGNED_CONTEXT((#81028))
GLOBAL_UNIT_ASSIGNED_CONTEXT((#81041,#81043,#81044))
REPRESENTATION_CONTEXT('','3D')
);
#81041=(
LENGTH_UNIT()
NAMED_UNIT(*)
SI_UNIT(.MILLI.,.METRE.)
);
#81043=(
NAMED_UNIT(*)
PLANE_ANGLE_UNIT()
SI_UNIT($,.RADIAN.)
);
#81044=(
NAMED_UNIT(*)
SI_UNIT($,.STERADIAN.)
SOLID_ANGLE_UNIT()
);
#81049=SHAPE_DEFINITION_REPRESENTATION(#81060,#81133);
#81060=PRODUCT_DEFINITION_SHAPE('',$,#81145);
#81133=SHAPE_REPRESENTATION('',(#15705),#81033);
#81140=PRODUCT_DEFINITION_CONTEXT('part definition',#81175,'design');
#81145=PRODUCT_DEFINITION('V-Way Roller Rail Base Side',
'V-Way Roller Rail Base Side',#81156,#81140);
#81156=PRODUCT_DEFINITION_FORMATION('',$,#81181);
#81175=APPLICATION_CONTEXT(
'Core Data for Automotive Mechanical Design Process');
#81176=PRODUCT_CONTEXT('part definition',#81175,'mechanical');
#81181=PRODUCT('V-Way Roller Rail Base Side',
'V-Way Roller Rail Base Side',$,(#81176));
#81192=PRESENTATION_STYLE_ASSIGNMENT((#81203));
#81203=SURFACE_STYLE_USAGE(.BOTH.,#81214);
#81214=SURFACE_SIDE_STYLE('',(#81225));
#81225=SURFACE_STYLE_FILL_AREA(#81236);
#81236=FILL_AREA_STYLE('Opaque(228,231,235)',(#81247));
#81247=FILL_AREA_STYLE_COLOUR('Opaque(228,231,235)',#81258);
#81258=COLOUR_RGB('Opaque(228,231,235)', 0.40784314, 0.44705882, 0.49803922);
ENDSEC;
END-ISO-10303-21;
